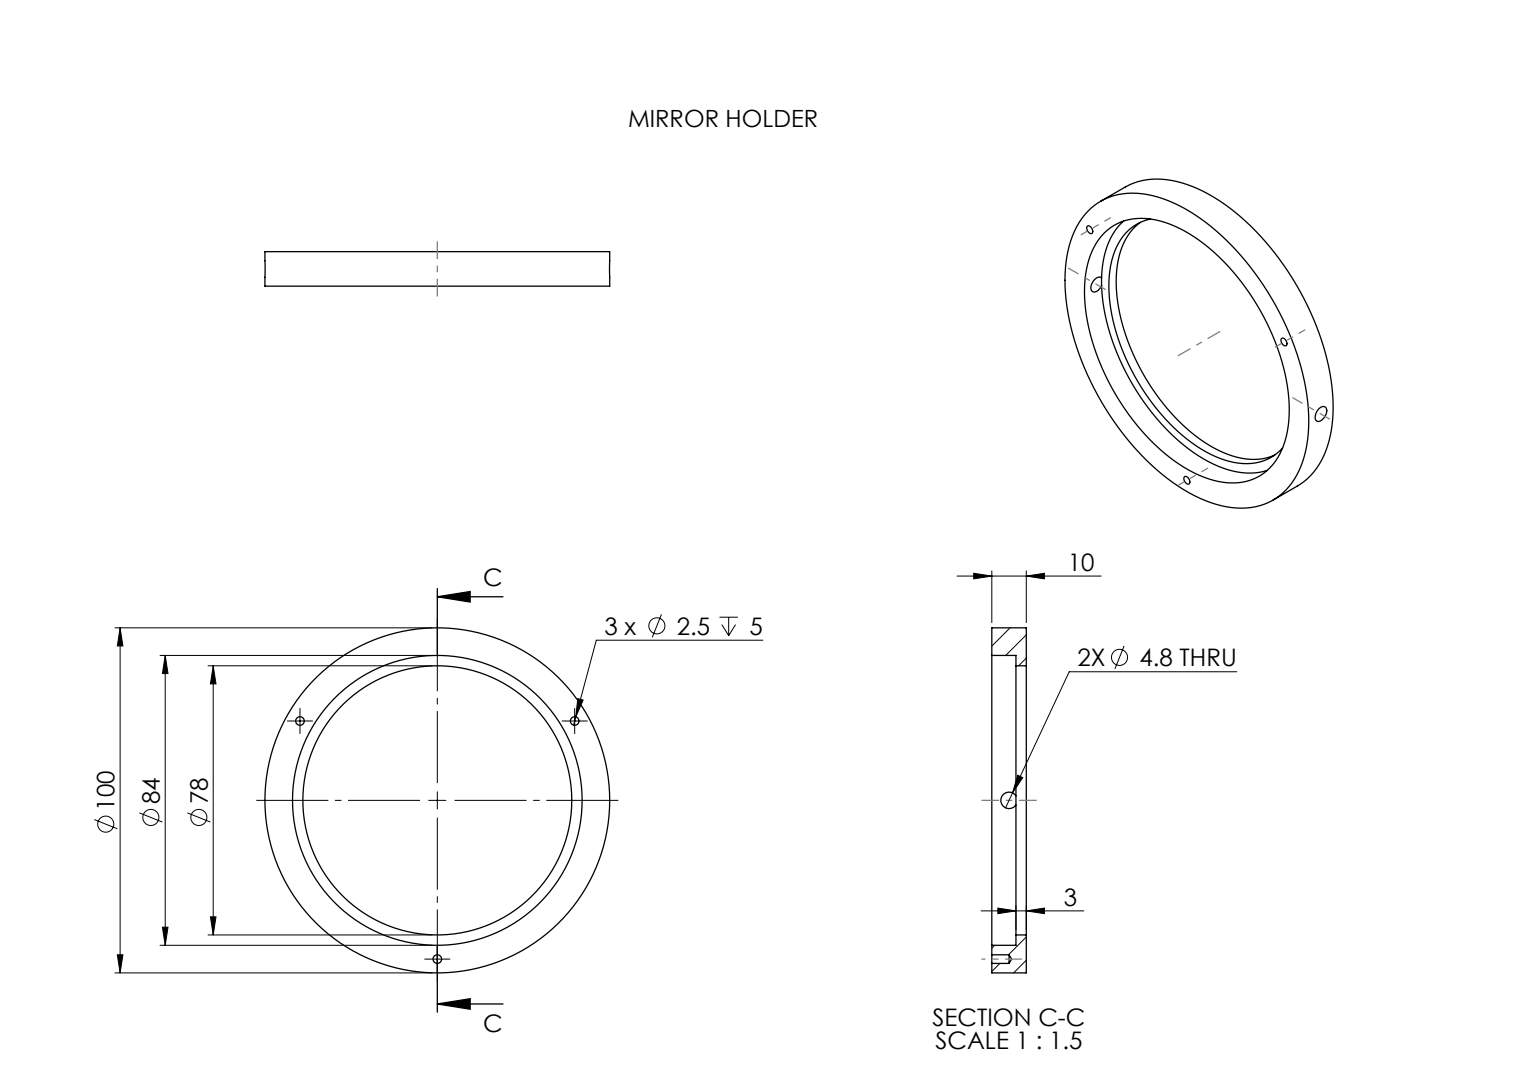
ISO-10303-21;
HEADER;
FILE_DESCRIPTION (('STEP AP214'),
    '1' );
FILE_NAME ('mirror holder.step',
    '2026-10-08T12:12:07',
    ( '' ),
    ( '' ),
    'SwSTEP 2.0',
    'SolidWorks 2026',
    '' );
FILE_SCHEMA (( 'AUTOMOTIVE_DESIGN' ));
ENDSEC;

DATA;
#6=DIRECTION ( 'NONE',  ( -1.000000000000000000, 0.000000000000000000, 0.000000000000000000 ) ) ;
#14=CARTESIAN_POINT ( 'NONE',  ( 49.97494079589864668, 83.41331875350536507, -1.807471472119508205 ) ) ;
#19=CARTESIAN_POINT ( 'NONE',  ( 42.00000000000004263, 84.74554347572708934, -2.399999999999959943 ) ) ;
#22=CYLINDRICAL_SURFACE ( 'NONE', #7576, 2.399999999999985256 ) ;
#23=ORIENTED_EDGE ( 'NONE', *, *, #1900, .T. ) ;
#31=VECTOR ( 'NONE', #6228, 1000.000000000000000 ) ;
#34=FACE_OUTER_BOUND ( 'NONE', #4042, .T. ) ;
#42=ORIENTED_EDGE ( 'NONE', *, *, #1737, .T. ) ;
#44=CARTESIAN_POINT ( 'NONE',  ( -42.00000000000000711, 85.00000000000046896, 2.399999999999971045 ) ) ;
#51=ORIENTED_EDGE ( 'NONE', *, *, #3552, .T. ) ;
#55=CARTESIAN_POINT ( 'NONE',  ( 41.93508307841050708, 82.66544186248239612, -0.5710001583723857133 ) ) ;
#57=ORIENTED_EDGE ( 'NONE', *, *, #5357, .F. ) ;
#58=DIRECTION ( 'NONE',  ( 1.412205397084881070E-17, -2.775557561562891967E-17, -1.000000000000000000 ) ) ;
#59=DIRECTION ( 'NONE',  ( -1.412205397084881070E-17, 2.775557561562891967E-17, 1.000000000000000000 ) ) ;
#71=B_SPLINE_CURVE_WITH_KNOTS ( 'NONE', 3,
 ( #3365, #3998, #818, #3718, #2730, #6286, #158, #589, #14, #5859, #6912, #2467, #2700, #6512, #1264, #1222, #4609, #1172, #6467, #3136, #4426, #5671, #1897, #8185, #2045, #5894, #631, #5007, #778, #5278, #552, #5630 ),
 .UNSPECIFIED., .F., .F.,
 ( 4, 2, 2, 2, 2, 2, 2, 2, 2, 2, 2, 2, 2, 2, 2, 4 ),
 ( 0.000000000000000000, 0.0004690358444888099608, 0.0009380716889776199215, 0.001407107533466429774, 0.001876143377955239843, 0.002345179222444049912, 0.002814215066932859548, 0.003752286755910464074, 0.004221322600399265469, 0.004690358444888067732, 0.005159394289376869995, 0.005628430133865671391, 0.006097465978354474521, 0.006566501822843276784, 0.007035537667332079914, 0.007504573511820881310 ),
 .UNSPECIFIED. ) ;
#72=ORIENTED_EDGE ( 'NONE', *, *, #716, .T. ) ;
#89=CARTESIAN_POINT ( 'NONE',  ( 41.93506701445378582, 87.33484857940398172, -0.5699281247695300312 ) ) ;
#90=DIRECTION ( 'NONE',  ( 0.000000000000000000, 0.000000000000000000, 1.000000000000000000 ) ) ;
#94=( GEOMETRIC_REPRESENTATION_CONTEXT ( 3 ) GLOBAL_UNCERTAINTY_ASSIGNED_CONTEXT ( ( #5253 ) ) GLOBAL_UNIT_ASSIGNED_CONTEXT ( ( #2108, #1487, #1650 ) ) REPRESENTATION_CONTEXT ( 'NONE', 'WORKASPACE' ) );
#108=AXIS2_PLACEMENT_3D ( 'NONE', #7357, #7319, #2957 ) ;
#116=AXIS2_PLACEMENT_3D ( 'NONE', #2904, #405, #2981 ) ;
#126=CARTESIAN_POINT ( 'NONE',  ( 39.00000000000003553, 85.00000000000017053, 2.000000000000043965 ) ) ;
#127=DIRECTION ( 'NONE',  ( -1.000000000000000000, 0.000000000000000000, 2.065146995210483462E-17 ) ) ;
#128=AXIS2_PLACEMENT_3D ( 'NONE', #4289, #6814, #1125 ) ;
#134=ORIENTED_EDGE ( 'NONE', *, *, #338, .F. ) ;
#138=CARTESIAN_POINT ( 'NONE',  ( 41.93122696811919070, 82.59745623955464566, -0.06342023833154092349 ) ) ;
#144=CARTESIAN_POINT ( 'NONE',  ( 5.930697612239895941E-15, 38.99999999999999289, -4.999999999999990230 ) ) ;
#146=CARTESIAN_POINT ( 'NONE',  ( -50.00000000000000711, 85.00000000000009948, -2.399999999999999467 ) ) ;
#150=EDGE_CURVE ( 'NONE', #5220, #7241, #7933, .T. ) ;
#152=CYLINDRICAL_SURFACE ( 'NONE', #1717, 39.00000000000002132 ) ;
#155=CARTESIAN_POINT ( 'NONE',  ( -50.00000000000000711, 85.00000000000009948, 5.000000000000045297 ) ) ;
#158=CARTESIAN_POINT ( 'NONE',  ( 49.98571321592399386, 83.79770962390523437, -2.083050663831888638 ) ) ;
#166=VERTEX_POINT ( 'NONE', #1074 ) ;
#176=DIRECTION ( 'NONE',  ( -1.000000000000000000, 0.000000000000000000, 1.412205397084726379E-17 ) ) ;
#192=ORIENTED_EDGE ( 'NONE', *, *, #1370, .F. ) ;
#201=EDGE_CURVE ( 'NONE', #2355, #5862, #1579, .T. ) ;
#202=DIRECTION ( 'NONE',  ( -1.000000000000000000, 0.000000000000000000, 1.032573497605241731E-17 ) ) ;
#213=STYLED_ITEM ( 'NONE', ( #3872 ), #6686 ) ;
#223=AXIS2_PLACEMENT_3D ( 'NONE', #6794, #1143, #8202 ) ;
#224=CARTESIAN_POINT ( 'NONE',  ( 41.97904239022140160, 83.67335008385828132, 2.000000000000015543 ) ) ;
#231=CIRCLE ( 'NONE', #4093, 50.00000000000002132 ) ;
#242=VECTOR ( 'NONE', #527, 1000.000000000000000 ) ;
#255=DIRECTION ( 'NONE',  ( 1.412205397084881070E-17, -2.775557561562891967E-17, -1.000000000000000000 ) ) ;
#278=DIRECTION ( 'NONE',  ( -1.000000000000000000, 0.000000000000000000, 0.000000000000000000 ) ) ;
#285=DIRECTION ( 'NONE',  ( 1.412205397084881070E-17, -2.775557561562891967E-17, -1.000000000000000000 ) ) ;
#296=FACE_OUTER_BOUND ( 'NONE', #3886, .T. ) ;
#306=CARTESIAN_POINT ( 'NONE',  ( -41.93238906222609330, 87.38229022169096538, 0.3178396967578642762 ) ) ;
#308=CARTESIAN_POINT ( 'NONE',  ( -49.94312129582967685, 82.61555530433810191, -0.3147289805187312162 ) ) ;
#310=FACE_BOUND ( 'NONE', #6643, .T. ) ;
#338=EDGE_CURVE ( 'NONE', #4916, #3085, #3906, .T. ) ;
#358=DIRECTION ( 'NONE',  ( 1.412205397084881070E-17, -2.775557561562891967E-17, -1.000000000000000000 ) ) ;
#363=AXIS2_PLACEMENT_3D ( 'NONE', #6847, #4450, #6938 ) ;
#373=AXIS2_PLACEMENT_3D ( 'NONE', #144, #3901, #4524 ) ;
#376=EDGE_LOOP ( 'NONE', ( #2346, #2970, #7740, #5830, #3828 ) ) ;
#377=AXIS2_PLACEMENT_3D ( 'NONE', #2206, #6560, #5374 ) ;
#392=CARTESIAN_POINT ( 'NONE',  ( -41.94721337724058685, 87.11014508430733372, -1.171319538143981820 ) ) ;
#403=ORIENTED_EDGE ( 'NONE', *, *, #5324, .F. ) ;
#405=DIRECTION ( 'NONE',  ( 1.412205397084881070E-17, -2.775557561562891967E-17, -1.000000000000000000 ) ) ;
#406=CARTESIAN_POINT ( 'NONE',  ( 1.270137496355039850E-14, 85.00000000000011369, 5.000000000000046185 ) ) ;
#411=EDGE_LOOP ( 'NONE', ( #6737, #422 ) ) ;
#419=ADVANCED_FACE ( 'NONE', ( #34 ), #2003, .T. ) ;
#422=ORIENTED_EDGE ( 'NONE', *, *, #7110, .F. ) ;
#423=CARTESIAN_POINT ( 'NONE',  ( 41.98518000931063199, 86.13243788719030647, 2.128825685961691416 ) ) ;
#425=SURFACE_SIDE_STYLE ('',( #7498 ) ) ;
#428=CARTESIAN_POINT ( 'NONE',  ( 50.00000000000002842, 85.15661249647209274, 2.399999999999996803 ) ) ;
#440=ORIENTED_EDGE ( 'NONE', *, *, #4363, .T. ) ;
#467=CARTESIAN_POINT ( 'NONE',  ( -41.93122500247569917, 82.59742185927619573, -0.06338927685520805155 ) ) ;
#468=( LENGTH_UNIT ( ) NAMED_UNIT ( * ) SI_UNIT ( .MILLI., .METRE. ) );
#479=VERTEX_POINT ( 'NONE', #3947 ) ;
#486=CARTESIAN_POINT ( 'NONE',  ( 1.274374112546295138E-14, 85.00000000000017053, 2.000000000000043521 ) ) ;
#493=VERTEX_POINT ( 'NONE', #7205 ) ;
#509=APPLICATION_CONTEXT ( 'automotive_design' ) ;
#513=CARTESIAN_POINT ( 'NONE',  ( -41.96846535023715319, 83.37031242132569275, -1.766478104244469272 ) ) ;
#518=ORIENTED_EDGE ( 'NONE', *, *, #6030, .F. ) ;
#527=DIRECTION ( 'NONE',  ( 1.412205397084881070E-17, -2.775557561562891967E-17, -1.000000000000000000 ) ) ;
#544=EDGE_LOOP ( 'NONE', ( #2163, #4537, #4576, #1786, #8039 ) ) ;
#552=CARTESIAN_POINT ( 'NONE',  ( 50.00000000000001421, 84.84335183244012057, 2.399999999999947509 ) ) ;
#557=CARTESIAN_POINT ( 'NONE',  ( -41.93910753963083948, 82.73888917238660667, -0.8146863085833027096 ) ) ;
#559=AXIS2_PLACEMENT_3D ( 'NONE', #4730, #358, #1076 ) ;
#570=PRODUCT_DEFINITION_FORMATION_WITH_SPECIFIED_SOURCE ( 'ANY', '', #3129, .NOT_KNOWN. ) ;
#578=CARTESIAN_POINT ( 'NONE',  ( 49.94601516505094452, 87.32303837806216507, 0.6228612347032452812 ) ) ;
#589=CARTESIAN_POINT ( 'NONE',  ( 49.97875682971463362, 83.53682071867390846, -1.908850074583744671 ) ) ;
#597=CARTESIAN_POINT ( 'NONE',  ( -41.96116023364841396, 83.19196313526902031, -1.583454828100236522 ) ) ;
#601=DIRECTION ( 'NONE',  ( 1.000000000000000000, 2.775557561562890365E-16, -1.734723475976806478E-17 ) ) ;
#611=B_SPLINE_CURVE_WITH_KNOTS ( 'NONE', 3,
 ( #7772, #6525, #3415, #4045, #1545, #3464 ),
 .UNSPECIFIED., .F., .F.,
 ( 4, 2, 4 ),
 ( 1.267684120349605325E-16, 0.0006999373991970426947, 0.001399874798393958755 ),
 .UNSPECIFIED. ) ;
#617=VECTOR ( 'NONE', #6433, 1000.000000000000114 ) ;
#619=EDGE_LOOP ( 'NONE', ( #2495, #2179, #7102, #6725 ) ) ;
#620=EDGE_CURVE ( 'NONE', #2013, #3227, #3446, .T. ) ;
#626=CARTESIAN_POINT ( 'NONE',  ( -41.98522237648275279, 83.86890273273840535, 2.129714952619055524 ) ) ;
#631=CARTESIAN_POINT ( 'NONE',  ( 49.98889375043669503, 83.93620601285596194, 2.157108981641731038 ) ) ;
#632=AXIS2_PLACEMENT_3D ( 'NONE', #7048, #58, #176 ) ;
#638=CARTESIAN_POINT ( 'NONE',  ( 41.98256188053848348, 83.77272253665795176, -2.078089480949315782 ) ) ;
#654=AXIS2_PLACEMENT_3D ( 'NONE', #1822, #7421, #1144 ) ;
#656=CARTESIAN_POINT ( 'NONE',  ( -50.00000000000000000, 85.31712395750685118, 2.400000000000064748 ) ) ;
#659=CIRCLE ( 'NONE', #7419, 42.00000000000002132 ) ;
#666=CARTESIAN_POINT ( 'NONE',  ( 49.97864901397263537, 86.46689848149799218, -1.906053348878814724 ) ) ;
#667=EDGE_CURVE ( 'NONE', #3060, #2355, #3891, .T. ) ;
#685=CARTESIAN_POINT ( 'NONE',  ( 41.95055335361874427, 82.96164397218471720, 1.273332678597350442 ) ) ;
#686=CARTESIAN_POINT ( 'NONE',  ( 39.00000000000003553, 85.00000000000017053, 5.000000000000047073 ) ) ;
#693=CARTESIAN_POINT ( 'NONE',  ( -49.95346081399732441, 87.15763333356271403, 1.062739361928057402 ) ) ;
#696=CARTESIAN_POINT ( 'NONE',  ( -50.00000000000000711, 85.00000000000009948, 5.000000000000047073 ) ) ;
#703=CARTESIAN_POINT ( 'NONE',  ( -49.97494079589861826, 83.41331875350518033, 1.807471472119332567 ) ) ;
#714=ORIENTED_EDGE ( 'NONE', *, *, #6444, .T. ) ;
#716=EDGE_CURVE ( 'NONE', #4997, #7730, #6980, .T. ) ;
#720=CARTESIAN_POINT ( 'NONE',  ( 41.97904239022140160, 83.67335008385828132, 2.000000000000015543 ) ) ;
#721=CARTESIAN_POINT ( 'NONE',  ( -59.99999999999999289, 85.00000000000045475, -1.387778780781445676E-14 ) ) ;
#732=CARTESIAN_POINT ( 'NONE',  ( 1.274374112546295138E-14, 85.00000000000017053, 2.000000000000043521 ) ) ;
#744=CARTESIAN_POINT ( 'NONE',  ( -42.00000000000000711, 85.00000000000011369, 2.000000000000043077 ) ) ;
#750=CARTESIAN_POINT ( 'NONE',  ( 41.96846535023716029, 86.62968757867487568, -1.766478104244785019 ) ) ;
#766=VECTOR ( 'NONE', #3845, 1000.000000000000000 ) ;
#778=CARTESIAN_POINT ( 'NONE',  ( 49.99635120648666486, 84.37668793019700786, 2.322944911472403451 ) ) ;
#790=CIRCLE ( 'NONE', #7560, 1.249999999999998668 ) ;
#795=AXIS2_PLACEMENT_3D ( 'NONE', #7855, #7230, #6693 ) ;
#798=CARTESIAN_POINT ( 'NONE',  ( 41.99105870351832692, 85.87498856589500917, -2.238438502733319790 ) ) ;
#807=CARTESIAN_POINT ( 'NONE',  ( -49.96357426530714463, 86.91018610273380318, 1.461418215542231058 ) ) ;
#818=CARTESIAN_POINT ( 'NONE',  ( 49.99924596088972351, 84.68545893936931179, -2.384433782424402182 ) ) ;
#820=EDGE_CURVE ( 'NONE', #7254, #5786, #2484, .T. ) ;
#829=ORIENTED_EDGE ( 'NONE', *, *, #2070, .F. ) ;
#842=CYLINDRICAL_SURFACE ( 'NONE', #373, 1.249999999999998446 ) ;
#844=FACE_OUTER_BOUND ( 'NONE', #6718, .T. ) ;
#872=CARTESIAN_POINT ( 'NONE',  ( 39.83716857408421674, 108.0000000000001421, 4.163336342344337027E-14 ) ) ;
#891=AXIS2_PLACEMENT_3D ( 'NONE', #5078, #7003, #1821 ) ;
#910=VERTEX_POINT ( 'NONE', #6172 ) ;
#913=CYLINDRICAL_SURFACE ( 'NONE', #7698, 50.00000000000002132 ) ;
#930=ORIENTED_EDGE ( 'NONE', *, *, #2930, .F. ) ;
#935=CARTESIAN_POINT ( 'NONE',  ( -41.93355926540179723, 87.36154593934628565, -0.4466446237679141396 ) ) ;
#940=LINE ( 'NONE', #5970, #5532 ) ;
#956=CARTESIAN_POINT ( 'NONE',  ( 50.00000000000003553, 85.00000000000012790, 5.000000000000047073 ) ) ;
#958=FACE_OUTER_BOUND ( 'NONE', #3987, .T. ) ;
#977=CARTESIAN_POINT ( 'NONE',  ( -41.95055335361870164, 87.03835602781624914, 1.273332678597377310 ) ) ;
#979=CARTESIAN_POINT ( 'NONE',  ( -49.95347202886236460, 82.84263588727921501, 1.063116165656198264 ) ) ;
#982=CARTESIAN_POINT ( 'NONE',  ( -42.00000000000000711, 85.00000000000011369, -2.399999999999999911 ) ) ;
#993=ORIENTED_EDGE ( 'NONE', *, *, #5499, .F. ) ;
#1001=CIRCLE ( 'NONE', #4066, 1.250000000000001110 ) ;
#1002=B_SPLINE_CURVE_WITH_KNOTS ( 'NONE', 3,
 ( #8152, #3001, #1732, #6920, #3636, #6787, #6161, #1814, #1135, #467, #5548, #4933, #6868, #557, #3677, #1180, #5638, #3772, #597, #513, #1772, #3140, #3052, #8114, #3729, #2433, #2303, #6251 ),
 .UNSPECIFIED., .F., .F.,
 ( 4, 2, 2, 2, 2, 2, 2, 2, 2, 2, 2, 2, 2, 4 ),
 ( 3.925231146709437917E-17, 0.0007633435184944741209, 0.001526687036988908994, 0.001908358796236126051, 0.002290030555483343541, 0.002671702314730560381, 0.003053374073977777655, 0.003435045833224994929, 0.003816717592472212203, 0.004198389351719429910, 0.004580061110966647184, 0.004961732870213864457, 0.005343404629461081731, 0.006106748147955515411 ),
 .UNSPECIFIED. ) ;
#1015=CARTESIAN_POINT ( 'NONE',  ( 41.08716857408421674, 108.0000000000001421, 4.161571085597980959E-14 ) ) ;
#1016=CARTESIAN_POINT ( 'NONE',  ( -41.97904239022133055, 86.32664991614245764, 2.000000000000043521 ) ) ;
#1048=ORIENTED_EDGE ( 'NONE', *, *, #8164, .F. ) ;
#1056=DIRECTION ( 'NONE',  ( 1.412205397084881070E-17, -2.775557561562891967E-17, -1.000000000000000000 ) ) ;
#1065=CARTESIAN_POINT ( 'NONE',  ( -49.98566918070725507, 83.79593159430156390, -2.081985610399898157 ) ) ;
#1070=ADVANCED_FACE ( 'NONE', ( #4597, #7827, #3384, #5307, #2141 ), #6617, .F. ) ;
#1074=CARTESIAN_POINT ( 'NONE',  ( 41.97904239022138029, 86.32664991614251448, 2.000000000000043521 ) ) ;
#1076=DIRECTION ( 'NONE',  ( -1.000000000000000000, 0.000000000000000000, 1.032573497605241731E-17 ) ) ;
#1080=ORIENTED_EDGE ( 'NONE', *, *, #6298, .T. ) ;
#1081=VERTEX_POINT ( 'NONE', #7286 ) ;
#1086=CIRCLE ( 'NONE', #559, 42.00000000000002132 ) ;
#1094=CYLINDRICAL_SURFACE ( 'NONE', #4649, 1.250000000000001110 ) ;
#1098=ADVANCED_FACE ( 'NONE', ( #844 ), #7167, .F. ) ;
#1103=CARTESIAN_POINT ( 'NONE',  ( -42.00000000000001421, 85.25445652427316645, -2.400000000000036326 ) ) ;
#1105=LINE ( 'NONE', #1196, #6872 ) ;
#1113=LINE ( 'NONE', #7561, #7414 ) ;
#1121=ORIENTED_EDGE ( 'NONE', *, *, #3316, .F. ) ;
#1125=DIRECTION ( 'NONE',  ( -1.000000000000000000, 0.000000000000000000, 1.412205397084881070E-17 ) ) ;
#1135=CARTESIAN_POINT ( 'NONE',  ( -41.93161960896017604, 82.60431869815872119, 0.1926422142525844872 ) ) ;
#1143=DIRECTION ( 'NONE',  ( 1.000000000000000000, 1.502586498047605218E-16, -1.412205397084881070E-17 ) ) ;
#1144=DIRECTION ( 'NONE',  ( -1.000000000000000000, 0.000000000000000000, 1.412205397084726379E-17 ) ) ;
#1164=CARTESIAN_POINT ( 'NONE',  ( 1.250000000000003997, 38.99999999999999289, 1.765256746356098409E-17 ) ) ;
#1170=AXIS2_PLACEMENT_3D ( 'NONE', #3288, #7106, #278 ) ;
#1172=CARTESIAN_POINT ( 'NONE',  ( 49.94600989915087297, 82.67684773840547052, 0.6225708050466158827 ) ) ;
#1178=AXIS2_PLACEMENT_3D ( 'NONE', #3683, #6835, #2439 ) ;
#1180=CARTESIAN_POINT ( 'NONE',  ( -41.94739886896328329, 82.89789273483425802, -1.165086683815163449 ) ) ;
#1190=ORIENTED_EDGE ( 'NONE', *, *, #7346, .T. ) ;
#1196=CARTESIAN_POINT ( 'NONE',  ( 42.00000000000003553, 85.00000000000012790, 5.000000000000045297 ) ) ;
#1210=ORIENTED_EDGE ( 'NONE', *, *, #4128, .T. ) ;
#1222=CARTESIAN_POINT ( 'NONE',  ( 49.94236411077207549, 82.59994436935576800, 0.1557065084606094330 ) ) ;
#1223=EDGE_LOOP ( 'NONE', ( #7509, #3451, #6070, #8010 ) ) ;
#1249=( GEOMETRIC_REPRESENTATION_CONTEXT ( 3 ) GLOBAL_UNCERTAINTY_ASSIGNED_CONTEXT ( ( #6118 ) ) GLOBAL_UNIT_ASSIGNED_CONTEXT ( ( #1271, #6870, #1733 ) ) REPRESENTATION_CONTEXT ( 'NONE', 'WORKASPACE' ) );
#1251=CARTESIAN_POINT ( 'NONE',  ( 49.96366046868875088, 86.90794461356699685, 1.464368789227024736 ) ) ;
#1256=PRODUCT_DEFINITION_CONTEXT ( 'detailed design', #509, 'design' ) ;
#1259=CARTESIAN_POINT ( 'NONE',  ( -41.99795150464620974, 84.52878598459807336, 2.364843771231078584 ) ) ;
#1264=CARTESIAN_POINT ( 'NONE',  ( 49.94237215279112263, 82.60011171831010302, -0.3139783802612605146 ) ) ;
#1265=ORIENTED_EDGE ( 'NONE', *, *, #1900, .F. ) ;
#1267=LINE ( 'NONE', #7624, #4912 ) ;
#1268=CARTESIAN_POINT ( 'NONE',  ( 41.97224931050730845, 83.45839738397258145, 1.857416509361046630 ) ) ;
#1270=ADVANCED_FACE ( 'NONE', ( #1773 ), #1094, .F. ) ;
#1271=( LENGTH_UNIT ( ) NAMED_UNIT ( * ) SI_UNIT ( .MILLI., .METRE. ) );
#1284=CARTESIAN_POINT ( 'NONE',  ( -49.99683717277851258, 85.63216245974585661, 2.336254100262071809 ) ) ;
#1296=CARTESIAN_POINT ( 'NONE',  ( 41.99057456900149532, 84.08235334355106261, 2.230005891995792133 ) ) ;
#1310=CARTESIAN_POINT ( 'NONE',  ( 41.93910753963084659, 87.26111082761428861, -0.8146863085835460705 ) ) ;
#1329=CARTESIAN_POINT ( 'NONE',  ( -39.00000000000000711, 85.00000000000017053, 5.000000000000045297 ) ) ;
#1333=DIRECTION ( 'NONE',  ( -1.000000000000000000, 0.000000000000000000, 2.065146995210483462E-17 ) ) ;
#1340=ADVANCED_FACE ( 'NONE', ( #7539 ), #22, .F. ) ;
#1350=EDGE_CURVE ( 'NONE', #4097, #5106, #4928, .T. ) ;
#1358=CARTESIAN_POINT ( 'NONE',  ( 41.93162413031729585, 82.60433940584233881, -0.1928755069450422688 ) ) ;
#1359=CYLINDRICAL_SURFACE ( 'NONE', #7664, 2.399999999999985256 ) ;
#1370=EDGE_CURVE ( 'NONE', #5556, #3085, #2015, .T. ) ;
#1371=CARTESIAN_POINT ( 'NONE',  ( -49.98886144361672734, 86.06516230458035466, 2.156352803700620768 ) ) ;
#1376=DIRECTION ( 'NONE',  ( 1.000000000000000000, 0.000000000000000000, -1.112002228190260397E-17 ) ) ;
#1398=LINE ( 'NONE', #7743, #5160 ) ;
#1406=CARTESIAN_POINT ( 'NONE',  ( -49.94817596271295201, 87.27669880683387760, -0.7754554817172341075 ) ) ;
#1416=ADVANCED_FACE ( 'NONE', ( #7818 ), #7120, .F. ) ;
#1427=PRODUCT_DEFINITION ( 'UNKNOWN', '', #570, #1256 ) ;
#1429=VERTEX_POINT ( 'NONE', #4670 ) ;
#1432=CARTESIAN_POINT ( 'NONE',  ( 41.94112359463814954, 82.77568671679536294, -0.9366119428080386111 ) ) ;
#1444=CIRCLE ( 'NONE', #5554, 1.249999999999998668 ) ;
#1447=EDGE_LOOP ( 'NONE', ( #6676, #192 ) ) ;
#1464=DIRECTION ( 'NONE',  ( -0.8571673007021118895, -1.430919794933844670E-16, -0.5150380749100549327 ) ) ;
#1466=EDGE_CURVE ( 'NONE', #7254, #493, #7769, .T. ) ;
#1481=DIRECTION ( 'NONE',  ( 1.412205397084881070E-17, -2.775557561562891967E-17, -1.000000000000000000 ) ) ;
#1483=DIRECTION ( 'NONE',  ( -1.000000000000000000, -1.502586498047605218E-16, 1.238733049487200360E-17 ) ) ;
#1487=( NAMED_UNIT ( * ) PLANE_ANGLE_UNIT ( ) SI_UNIT ( $, .RADIAN. ) );
#1497=ORIENTED_EDGE ( 'NONE', *, *, #7301, .T. ) ;
#1502=FACE_OUTER_BOUND ( 'NONE', #6197, .T. ) ;
#1512=DIRECTION ( 'NONE',  ( 1.412205397084881070E-17, -2.775557561562891967E-17, -1.000000000000000000 ) ) ;
#1515=DIRECTION ( 'NONE',  ( -1.000000000000000000, 0.000000000000000000, 0.000000000000000000 ) ) ;
#1517=CARTESIAN_POINT ( 'NONE',  ( -59.99999999999999289, 85.00000000000045475, -1.387778780781445676E-14 ) ) ;
#1536=LINE ( 'NONE', #6474, #4626 ) ;
#1545=CARTESIAN_POINT ( 'NONE',  ( -41.98520465537847457, 86.13165801428257851, 2.129342995125455662 ) ) ;
#1553=ADVANCED_FACE ( 'NONE', ( #5418 ), #7935, .T. ) ;
#1559=ORIENTED_EDGE ( 'NONE', *, *, #7278, .F. ) ;
#1561=CONICAL_SURFACE ( 'NONE', #3019, 1.249999999999998002, 1.029744258676653645 ) ;
#1566=ADVANCED_FACE ( 'NONE', ( #1641 ), #6697, .F. ) ;
#1569=CIRCLE ( 'NONE', #363, 50.00000000000002132 ) ;
#1579=CIRCLE ( 'NONE', #5829, 42.00000000000002132 ) ;
#1587=AXIS2_PLACEMENT_3D ( 'NONE', #3942, #5152, #6454 ) ;
#1598=EDGE_CURVE ( 'NONE', #5786, #1081, #7237, .T. ) ;
#1600=DIRECTION ( 'NONE',  ( -1.000000000000000000, 0.000000000000000000, 0.000000000000000000 ) ) ;
#1601=CIRCLE ( 'NONE', #795, 39.00000000000002132 ) ;
#1622=DIRECTION ( 'NONE',  ( 1.000000000000000000, 1.502586498047605218E-16, -1.412205397084881070E-17 ) ) ;
#1630=EDGE_CURVE ( 'NONE', #7075, #7290, #71, .T. ) ;
#1641=FACE_OUTER_BOUND ( 'NONE', #2635, .T. ) ;
#1647=EDGE_CURVE ( 'NONE', #7219, #5129, #1001, .T. ) ;
#1650=( NAMED_UNIT ( * ) SI_UNIT ( $, .STERADIAN. ) SOLID_ANGLE_UNIT ( ) );
#1654=CARTESIAN_POINT ( 'NONE',  ( -49.99423685432763875, 84.22705925652886094, -2.277573141052998462 ) ) ;
#1671=DIRECTION ( 'NONE',  ( 1.000000000000000000, 1.502586498047605218E-16, -1.412205397084881070E-17 ) ) ;
#1672=CARTESIAN_POINT ( 'NONE',  ( -41.08716857408418122, 108.0000000000001990, -4.999999999999976907 ) ) ;
#1687=ORIENTED_EDGE ( 'NONE', *, *, #7096, .T. ) ;
#1692=CARTESIAN_POINT ( 'NONE',  ( -41.97904239022133055, 86.32664991614245764, 2.000000000000043521 ) ) ;
#1711=EDGE_LOOP ( 'NONE', ( #4384, #23, #2821 ) ) ;
#1717=AXIS2_PLACEMENT_3D ( 'NONE', #732, #5741, #1376 ) ;
#1726=AXIS2_PLACEMENT_3D ( 'NONE', #5818, #5131, #6438 ) ;
#1732=CARTESIAN_POINT ( 'NONE',  ( -41.96471864142489494, 83.27150586048362868, 1.684781847096441298 ) ) ;
#1733=( NAMED_UNIT ( * ) SI_UNIT ( $, .STERADIAN. ) SOLID_ANGLE_UNIT ( ) );
#1737=EDGE_CURVE ( 'NONE', #1769, #4916, #940, .T. ) ;
#1742=CYLINDRICAL_SURFACE ( 'NONE', #223, 2.399999999999985256 ) ;
#1744=DIRECTION ( 'NONE',  ( 1.412205397084881070E-17, -2.775557561562891967E-17, -1.000000000000000000 ) ) ;
#1756=CARTESIAN_POINT ( 'NONE',  ( 49.94311118432961649, 87.38465289139496406, -0.3128412141714160266 ) ) ;
#1762=DIRECTION ( 'NONE',  ( 1.412205397084881070E-17, -2.775557561562891967E-17, -1.000000000000000000 ) ) ;
#1764=FACE_OUTER_BOUND ( 'NONE', #2988, .T. ) ;
#1767=DIRECTION ( 'NONE',  ( -1.000000000000000000, 0.000000000000000000, 2.065146995210483462E-17 ) ) ;
#1769=VERTEX_POINT ( 'NONE', #982 ) ;
#1772=CARTESIAN_POINT ( 'NONE',  ( -41.97210380486418302, 83.46605959390291218, -1.850206309317909303 ) ) ;
#1773=FACE_OUTER_BOUND ( 'NONE', #6146, .T. ) ;
#1786=ORIENTED_EDGE ( 'NONE', *, *, #4520, .T. ) ;
#1792=CARTESIAN_POINT ( 'NONE',  ( -39.00000000000000711, 85.00000000000017053, 2.000000000000043965 ) ) ;
#1793=DIRECTION ( 'NONE',  ( -1.412205397084881070E-17, 2.775557561562891967E-17, 1.000000000000000000 ) ) ;
#1800=EDGE_LOOP ( 'NONE', ( #1919, #2477, #6514, #4664 ) ) ;
#1801=ORIENTED_EDGE ( 'NONE', *, *, #3973, .T. ) ;
#1814=CARTESIAN_POINT ( 'NONE',  ( -41.93240078214817856, 82.61791640338877585, 0.3192077737422600037 ) ) ;
#1818=ORIENTED_EDGE ( 'NONE', *, *, #6302, .F. ) ;
#1821=DIRECTION ( 'NONE',  ( -1.000000000000000000, 0.000000000000000000, 1.032573497605241731E-17 ) ) ;
#1822=CARTESIAN_POINT ( 'NONE',  ( -39.83716857408418122, 108.0000000000001421, 4.163336342344337027E-14 ) ) ;
#1834=CARTESIAN_POINT ( 'NONE',  ( 49.99422766321050204, 85.77334557296516948, 2.277359159638543851 ) ) ;
#1861=CARTESIAN_POINT ( 'NONE',  ( -42.00000000000000711, 85.00000000000046896, 2.399999999999971045 ) ) ;
#1864=DIRECTION ( 'NONE',  ( 1.000000000000000000, 2.775557561562890365E-16, -1.734723475976806478E-17 ) ) ;
#1870=CYLINDRICAL_SURFACE ( 'NONE', #5302, 39.00000000000002132 ) ;
#1873=VECTOR ( 'NONE', #1744, 1000.000000000000000 ) ;
#1877=AXIS2_PLACEMENT_3D ( 'NONE', #6386, #5148, #601 ) ;
#1888=CARTESIAN_POINT ( 'NONE',  ( 41.97904239022140160, 83.67335008385828132, 2.000000000000015543 ) ) ;
#1892=FACE_OUTER_BOUND ( 'NONE', #1223, .T. ) ;
#1897=CARTESIAN_POINT ( 'NONE',  ( 49.96737414687255097, 83.19055800108181131, 1.584620125915989775 ) ) ;
#1900=EDGE_CURVE ( 'NONE', #7604, #5220, #7469, .T. ) ;
#1904=CARTESIAN_POINT ( 'NONE',  ( 41.96864087686234512, 83.36448938425077415, -1.774759388939936899 ) ) ;
#1911=ORIENTED_EDGE ( 'NONE', *, *, #6672, .F. ) ;
#1919=ORIENTED_EDGE ( 'NONE', *, *, #1466, .F. ) ;
#1926=CARTESIAN_POINT ( 'NONE',  ( 50.00000000000004974, 85.31712395750716382, -2.400000000000014566 ) ) ;
#1944=CARTESIAN_POINT ( 'NONE',  ( 42.00000000000003553, 85.00000000000012790, -2.399999999999999023 ) ) ;
#1950=DIRECTION ( 'NONE',  ( 1.412205397084881070E-17, -2.775557561562891967E-17, -1.000000000000000000 ) ) ;
#1963=CARTESIAN_POINT ( 'NONE',  ( -49.99924596088969508, 84.68545893936895652, 2.384433782424337789 ) ) ;
#1968=ORIENTED_EDGE ( 'NONE', *, *, #7077, .F. ) ;
#1981=CARTESIAN_POINT ( 'NONE',  ( 41.93161561614421373, 82.60424888756949713, 0.1913511295313893579 ) ) ;
#1997=CARTESIAN_POINT ( 'NONE',  ( -49.94313152867111683, 87.38422970439138737, -0.3160888171752656572 ) ) ;
#2001=ORIENTED_EDGE ( 'NONE', *, *, #7821, .F. ) ;
#2002=AXIS2_PLACEMENT_3D ( 'NONE', #4200, #1762, #6191 ) ;
#2003=CYLINDRICAL_SURFACE ( 'NONE', #6823, 42.00000000000002132 ) ;
#2013=VERTEX_POINT ( 'NONE', #1329 ) ;
#2015=CIRCLE ( 'NONE', #1877, 50.00000000000002132 ) ;
#2017=CARTESIAN_POINT ( 'NONE',  ( -38.58716857408418122, 108.0000000000001990, -4.999999999999976907 ) ) ;
#2025=DIRECTION ( 'NONE',  ( 1.412205397084881070E-17, -2.775557561562891967E-17, -1.000000000000000000 ) ) ;
#2026=CARTESIAN_POINT ( 'NONE',  ( 42.00000000000003553, 85.00000000000012790, -2.399999999999999023 ) ) ;
#2039=DIRECTION ( 'NONE',  ( 1.412205397084881070E-17, -2.775557561562891967E-17, -1.000000000000000000 ) ) ;
#2045=CARTESIAN_POINT ( 'NONE',  ( 49.97873132679187336, 83.53599209938494141, 1.908173386893731616 ) ) ;
#2059=CARTESIAN_POINT ( 'NONE',  ( 41.93240078214817146, 87.38208359661221891, 0.3192077737421512018 ) ) ;
#2064=DIRECTION ( 'NONE',  ( 1.412205397084881070E-17, -2.775557561562891967E-17, -1.000000000000000000 ) ) ;
#2070=EDGE_CURVE ( 'NONE', #4916, #1429, #3080, .T. ) ;
#2079=AXIS2_PLACEMENT_3D ( 'NONE', #6156, #3544, #6821 ) ;
#2102=CIRCLE ( 'NONE', #891, 42.00000000000002132 ) ;
#2104=CIRCLE ( 'NONE', #6349, 42.00000000000002132 ) ;
#2108=( LENGTH_UNIT ( ) NAMED_UNIT ( * ) SI_UNIT ( .MILLI., .METRE. ) );
#2126=VECTOR ( 'NONE', #5355, 1000.000000000000000 ) ;
#2141=FACE_BOUND ( 'NONE', #3104, .T. ) ;
#2149=CARTESIAN_POINT ( 'NONE',  ( -49.95667649488481032, 82.91716997302802383, 1.202799388691194959 ) ) ;
#2163=ORIENTED_EDGE ( 'NONE', *, *, #6444, .F. ) ;
#2173=LINE ( 'NONE', #4130, #7287 ) ;
#2179=ORIENTED_EDGE ( 'NONE', *, *, #2648, .T. ) ;
#2188=CARTESIAN_POINT ( 'NONE',  ( 1.274374112546295138E-14, 85.00000000000017053, 2.000000000000043521 ) ) ;
#2206=CARTESIAN_POINT ( 'NONE',  ( -39.83716857408418122, 108.0000000000001990, -4.999999999999976907 ) ) ;
#2226=CARTESIAN_POINT ( 'NONE',  ( -49.97498335796541369, 83.41456698278581428, -1.808729786019619423 ) ) ;
#2231=ORIENTED_EDGE ( 'NONE', *, *, #5399, .T. ) ;
#2236=AXIS2_PLACEMENT_3D ( 'NONE', #3540, #4202, #6778 ) ;
#2242=CARTESIAN_POINT ( 'NONE',  ( -41.08716857408418122, 108.0000000000001990, -4.999999999999976907 ) ) ;
#2246=PRODUCT_CONTEXT ( 'NONE', #7736, 'mechanical' ) ;
#2255=AXIS2_PLACEMENT_3D ( 'NONE', #4020, #255, #6032 ) ;
#2267=ORIENTED_EDGE ( 'NONE', *, *, #2993, .T. ) ;
#2273=LINE ( 'NONE', #6711, #6943 ) ;
#2302=CARTESIAN_POINT ( 'NONE',  ( 41.97904239022138029, 86.32664991614251448, 2.000000000000043521 ) ) ;
#2303=CARTESIAN_POINT ( 'NONE',  ( -42.00000000000001421, 84.74546678807557498, -2.399999999999965272 ) ) ;
#2308=EDGE_LOOP ( 'NONE', ( #1818, #5430, #1801, #6222, #3675, #134, #6812, #7886 ) ) ;
#2311=CARTESIAN_POINT ( 'NONE',  ( -42.00000000000000711, 85.00000000000011369, -2.399999999999999911 ) ) ;
#2334=DIRECTION ( 'NONE',  ( 1.412205397084881070E-17, -2.775557561562891967E-17, -1.000000000000000000 ) ) ;
#2346=ORIENTED_EDGE ( 'NONE', *, *, #2525, .T. ) ;
#2348=CARTESIAN_POINT ( 'NONE',  ( -41.95400501379501890, 86.96664633062719929, 1.381527937806870998 ) ) ;
#2349=DIRECTION ( 'NONE',  ( -1.000000000000000000, -1.502586498047605218E-16, 1.238733049487200360E-17 ) ) ;
#2350=DIRECTION ( 'NONE',  ( 1.412205397084881070E-17, -2.775557561562891967E-17, -1.000000000000000000 ) ) ;
#2355=VERTEX_POINT ( 'NONE', #224 ) ;
#2363=CARTESIAN_POINT ( 'NONE',  ( -42.00000000000000711, 85.00000000000011369, -5.000000000000005329 ) ) ;
#2373=ORIENTED_EDGE ( 'NONE', *, *, #5785, .T. ) ;
#2386=CIRCLE ( 'NONE', #377, 1.250000000000001110 ) ;
#2389=ADVANCED_FACE ( 'NONE', ( #3444 ), #7320, .F. ) ;
#2396=AXIS2_PLACEMENT_3D ( 'NONE', #2569, #5111, #1864 ) ;
#2433=CARTESIAN_POINT ( 'NONE',  ( -41.99757081983619145, 84.48764332354225814, -2.358461006662856185 ) ) ;
#2439=DIRECTION ( 'NONE',  ( -1.000000000000000000, 0.000000000000000000, 1.412205397084726379E-17 ) ) ;
#2452=DIRECTION ( 'NONE',  ( 1.412205397084881070E-17, -2.775557561562891967E-17, -1.000000000000000000 ) ) ;
#2457=ADVANCED_FACE ( 'NONE', ( #7872, #310 ), #7837, .T. ) ;
#2467=CARTESIAN_POINT ( 'NONE',  ( 49.95667649488486717, 82.91716997302819436, -1.202799388691395910 ) ) ;
#2477=ORIENTED_EDGE ( 'NONE', *, *, #820, .T. ) ;
#2484=LINE ( 'NONE', #6218, #242 ) ;
#2493=CARTESIAN_POINT ( 'NONE',  ( 49.97874610126637407, 86.47445480916304916, 1.919346332466817406 ) ) ;
#2495=ORIENTED_EDGE ( 'NONE', *, *, #7453, .T. ) ;
#2498=ORIENTED_EDGE ( 'NONE', *, *, #7821, .T. ) ;
#2517=CARTESIAN_POINT ( 'NONE',  ( 41.96116023364841396, 86.80803686473167602, -1.583454828100570255 ) ) ;
#2519=PRESENTATION_STYLE_ASSIGNMENT (( #6295 ) ) ;
#2525=EDGE_CURVE ( 'NONE', #166, #2355, #1086, .T. ) ;
#2527=ORIENTED_EDGE ( 'NONE', *, *, #667, .T. ) ;
#2548=CARTESIAN_POINT ( 'NONE',  ( 49.96738998307159818, 86.80892218194638588, -1.585032901986132226 ) ) ;
#2552=CARTESIAN_POINT ( 'NONE',  ( 41.99758845363990645, 84.53527270025752216, 2.357482664457419830 ) ) ;
#2567=AXIS2_PLACEMENT_3D ( 'NONE', #4143, #5319, #4687 ) ;
#2569=CARTESIAN_POINT ( 'NONE',  ( 1.270137496355039850E-14, 85.00000000000011369, 5.000000000000046185 ) ) ;
#2578=CARTESIAN_POINT ( 'NONE',  ( -49.94236053903777162, 87.40012995604533330, 0.1563225272305456826 ) ) ;
#2583=( GEOMETRIC_REPRESENTATION_CONTEXT ( 3 ) GLOBAL_UNCERTAINTY_ASSIGNED_CONTEXT ( ( #8018 ) ) GLOBAL_UNIT_ASSIGNED_CONTEXT ( ( #468, #3002, #5014 ) ) REPRESENTATION_CONTEXT ( 'NONE', 'WORKASPACE' ) );
#2610=CARTESIAN_POINT ( 'NONE',  ( 50.00000000000003553, 85.00000000000012790, 5.000000000000045297 ) ) ;
#2618=LINE ( 'NONE', #7642, #617 ) ;
#2635=EDGE_LOOP ( 'NONE', ( #5794, #6445, #51, #3105 ) ) ;
#2637=CARTESIAN_POINT ( 'NONE',  ( 41.96471864142488073, 86.72849413951723818, 1.684781847096518792 ) ) ;
#2640=VECTOR ( 'NONE', #3843, 1000.000000000000114 ) ;
#2648=EDGE_CURVE ( 'NONE', #4584, #2013, #3077, .T. ) ;
#2654=CARTESIAN_POINT ( 'NONE',  ( -49.97864901397259985, 86.46689848149772217, 1.906053348878929077 ) ) ;
#2661=FACE_OUTER_BOUND ( 'NONE', #8158, .T. ) ;
#2670=ORIENTED_EDGE ( 'NONE', *, *, #2525, .F. ) ;
#2678=CARTESIAN_POINT ( 'NONE',  ( 41.93504501510003735, 82.66492853475577363, 0.5690079308735644936 ) ) ;
#2679=CARTESIAN_POINT ( 'NONE',  ( -39.83716857408418122, 108.0000000000001421, 4.163336342344337027E-14 ) ) ;
#2683=EDGE_CURVE ( 'NONE', #5862, #7730, #6790, .T. ) ;
#2700=CARTESIAN_POINT ( 'NONE',  ( 49.95347202886240012, 82.84263588727935712, -1.063116165656391221 ) ) ;
#2703=MECHANICAL_DESIGN_GEOMETRIC_PRESENTATION_REPRESENTATION('',(#6950),#2583);
#2725=CYLINDRICAL_SURFACE ( 'NONE', #6206, 42.00000000000002132 ) ;
#2730=CARTESIAN_POINT ( 'NONE',  ( 49.99422363137632885, 84.22622254513471773, -2.277283319317807031 ) ) ;
#2746=ORIENTED_EDGE ( 'NONE', *, *, #7323, .F. ) ;
#2753=CARTESIAN_POINT ( 'NONE',  ( 39.83716857408421674, 108.0000000000001990, -4.999999999999976907 ) ) ;
#2758=CYLINDRICAL_SURFACE ( 'NONE', #2255, 1.249999999999998446 ) ;
#2791=ORIENTED_EDGE ( 'NONE', *, *, #5357, .T. ) ;
#2795=DIRECTION ( 'NONE',  ( 1.412205397084881070E-17, -2.775557561562891967E-17, -1.000000000000000000 ) ) ;
#2798=DIRECTION ( 'NONE',  ( 1.412205397084881070E-17, -2.775557561562891967E-17, -1.000000000000000000 ) ) ;
#2813=CARTESIAN_POINT ( 'NONE',  ( -41.94160807294379367, 87.21436019787591931, 0.9342823132686582932 ) ) ;
#2821=ORIENTED_EDGE ( 'NONE', *, *, #150, .T. ) ;
#2841=DIRECTION ( 'NONE',  ( -1.000000000000000000, 0.000000000000000000, 1.412205397084726379E-17 ) ) ;
#2851=DIRECTION ( 'NONE',  ( -1.000000000000000000, 0.000000000000000000, 0.000000000000000000 ) ) ;
#2853=CARTESIAN_POINT ( 'NONE',  ( -49.95669240716469517, 82.91758674606776935, -1.203334160065746339 ) ) ;
#2854=DIRECTION ( 'NONE',  ( -1.000000000000000000, -1.502586498047605218E-16, 1.412205397084881070E-17 ) ) ;
#2868=AXIS2_PLACEMENT_3D ( 'NONE', #3767, #5717, #3332 ) ;
#2874=ORIENTED_EDGE ( 'NONE', *, *, #2683, .F. ) ;
#2891=LINE ( 'NONE', #1015, #4865 ) ;
#2894=CARTESIAN_POINT ( 'NONE',  ( -49.94600989915083744, 82.67684773840545631, -0.6225708050467673171 ) ) ;
#2904=CARTESIAN_POINT ( 'NONE',  ( 5.860087342385653250E-15, 38.99999999999999289, 0.000000000000000000 ) ) ;
#2905=CIRCLE ( 'NONE', #5045, 42.00000000000002132 ) ;
#2918=VECTOR ( 'NONE', #4201, 1000.000000000000000 ) ;
#2920=ORIENTED_EDGE ( 'NONE', *, *, #6168, .F. ) ;
#2925=AXIS2_PLACEMENT_3D ( 'NONE', #1517, #1483, #5345 ) ;
#2930=EDGE_CURVE ( 'NONE', #479, #5129, #2618, .T. ) ;
#2937=CARTESIAN_POINT ( 'NONE',  ( -41.93161561614412847, 87.39575111243146921, 0.1913511295312773086 ) ) ;
#2941=ORIENTED_EDGE ( 'NONE', *, *, #4363, .F. ) ;
#2946=DIRECTION ( 'NONE',  ( 1.000000000000000000, 2.775557561562890365E-16, -1.734723475976806478E-17 ) ) ;
#2957=DIRECTION ( 'NONE',  ( -1.000000000000000000, 0.000000000000000000, 2.065146995210483462E-17 ) ) ;
#2964=CARTESIAN_POINT ( 'NONE',  ( 42.00000000000003553, 85.00000000000049738, 2.399999999999971934 ) ) ;
#2970=ORIENTED_EDGE ( 'NONE', *, *, #201, .T. ) ;
#2973=CARTESIAN_POINT ( 'NONE',  ( -41.93508307841045024, 87.33455813751852759, -0.5710001583726183050 ) ) ;
#2975=LINE ( 'NONE', #5519, #1873 ) ;
#2981=DIRECTION ( 'NONE',  ( -1.000000000000000000, 0.000000000000000000, 1.412205397084881070E-17 ) ) ;
#2988=EDGE_LOOP ( 'NONE', ( #7756, #8019, #6112, #1210, #7036, #7651, #1121, #3848 ) ) ;
#2993=EDGE_CURVE ( 'NONE', #4127, #7254, #2891, .T. ) ;
#3001=CARTESIAN_POINT ( 'NONE',  ( -41.97224725382100274, 83.45833230446734774, 1.857373340501012660 ) ) ;
#3002=( NAMED_UNIT ( * ) PLANE_ANGLE_UNIT ( ) SI_UNIT ( $, .RADIAN. ) );
#3019=AXIS2_PLACEMENT_3D ( 'NONE', #7184, #5174, #7070 ) ;
#3020=ORIENTED_EDGE ( 'NONE', *, *, #4793, .T. ) ;
#3024=DIRECTION ( 'NONE',  ( -1.000000000000000000, 0.000000000000000000, 1.032573497605241731E-17 ) ) ;
#3036=ORIENTED_EDGE ( 'NONE', *, *, #2993, .F. ) ;
#3050=CIRCLE ( 'NONE', #7569, 1.250000000000001110 ) ;
#3052=CARTESIAN_POINT ( 'NONE',  ( -41.98244464128907794, 83.78046611586739800, -2.071021427375471902 ) ) ;
#3060=VERTEX_POINT ( 'NONE', #6577 ) ;
#3073=EDGE_LOOP ( 'NONE', ( #4827, #714, #6402, #6165, #1497 ) ) ;
#3077=LINE ( 'NONE', #1792, #31 ) ;
#3079=CARTESIAN_POINT ( 'NONE',  ( 49.97491191256678178, 86.58758952878010007, -1.806678789609242664 ) ) ;
#3080=B_SPLINE_CURVE_WITH_KNOTS ( 'NONE', 3,
 ( #146, #3869, #5234, #5120, #7089, #6395, #3904, #4598, #6428, #3986, #5082, #1406, #3240, #1997, #4483, #2578, #4528, #6503, #7602, #693, #7052, #807, #6350, #3944, #2654, #6968, #1371, #1284, #656, #3205 ),
 .UNSPECIFIED., .F., .F.,
 ( 4, 2, 2, 2, 2, 2, 2, 2, 2, 2, 2, 2, 2, 2, 4 ),
 ( 0.007504573511820675745, 0.007973502549960232236, 0.008442431588099789594, 0.009380289664378940739, 0.009849218702518501567, 0.01031814774065806413, 0.01078707677879762669, 0.01125600581693718752, 0.01172493485507674835, 0.01219386389321631091, 0.01266279293135587347, 0.01313172196949543430, 0.01360065100763499513, 0.01406958004577455595, 0.01500743812205367934 ),
 .UNSPECIFIED. ) ;
#3085=VERTEX_POINT ( 'NONE', #7867 ) ;
#3086=DIRECTION ( 'NONE',  ( 1.412205397084881070E-17, -2.775557561562891967E-17, -1.000000000000000000 ) ) ;
#3096=CARTESIAN_POINT ( 'NONE',  ( 50.00000000000003553, 85.00000000000012790, 2.399999999999971489 ) ) ;
#3098=FILL_AREA_STYLE_COLOUR ( '', #5883 ) ;
#3104=EDGE_LOOP ( 'NONE', ( #2373, #4277 ) ) ;
#3105=ORIENTED_EDGE ( 'NONE', *, *, #5324, .T. ) ;
#3121=CARTESIAN_POINT ( 'NONE',  ( 49.99637443241782364, 85.62167278847336149, 2.323444847100735178 ) ) ;
#3129=PRODUCT ( 'mirror holder', 'mirror holder', '', ( #2246 ) ) ;
#3136=CARTESIAN_POINT ( 'NONE',  ( 49.95346277782375921, 82.84241399044236687, 1.062802698623439568 ) ) ;
#3140=CARTESIAN_POINT ( 'NONE',  ( -41.97907998747121638, 83.67059623091998333, -2.002229301367134617 ) ) ;
#3162=CARTESIAN_POINT ( 'NONE',  ( 41.08716857408421674, 108.0000000000001990, -4.999999999999976907 ) ) ;
#3164=CARTESIAN_POINT ( 'NONE',  ( 49.94237310791758944, 87.39986840612067454, 0.1602877778558433053 ) ) ;
#3167=AXIS2_PLACEMENT_3D ( 'NONE', #2679, #2798, #3302 ) ;
#3171=CIRCLE ( 'NONE', #632, 1.250000000000001110 ) ;
#3189=CARTESIAN_POINT ( 'NONE',  ( 41.94160807294385762, 82.78563980212508966, 0.9342823132686682852 ) ) ;
#3194=CIRCLE ( 'NONE', #5191, 39.00000000000002132 ) ;
#3196=ORIENTED_EDGE ( 'NONE', *, *, #4960, .T. ) ;
#3205=CARTESIAN_POINT ( 'NONE',  ( -49.99999999999999289, 85.00000000000005684, 2.400000000000013234 ) ) ;
#3213=CARTESIAN_POINT ( 'NONE',  ( 49.94597403161979798, 87.32391958025814915, -0.6195456578939724235 ) ) ;
#3216=DIRECTION ( 'NONE',  ( 1.412205397084881070E-17, -2.775557561562891967E-17, -1.000000000000000000 ) ) ;
#3227=VERTEX_POINT ( 'NONE', #686 ) ;
#3231=CARTESIAN_POINT ( 'NONE',  ( 41.95042219981620235, 87.04630884801559887, 1.280157006458500613 ) ) ;
#3233=AXIS2_PLACEMENT_3D ( 'NONE', #486, #2452, #3024 ) ;
#3236=ADVANCED_FACE ( 'NONE', ( #4515 ), #1359, .F. ) ;
#3240=CARTESIAN_POINT ( 'NONE',  ( -49.94601516505092320, 87.32303837806215085, -0.6228612347031499130 ) ) ;
#3248=CARTESIAN_POINT ( 'NONE',  ( -49.96742166427387843, 83.19195211451609850, 1.586024383261720239 ) ) ;
#3252=CARTESIAN_POINT ( 'NONE',  ( 41.99613340007108064, 84.41915023570773258, 2.331601159595727779 ) ) ;
#3254=ORIENTED_EDGE ( 'NONE', *, *, #7110, .T. ) ;
#3267=CARTESIAN_POINT ( 'NONE',  ( 41.93355926540186118, 82.63845406065466648, -0.4466446237676945930 ) ) ;
#3288=CARTESIAN_POINT ( 'NONE',  ( -39.83716857408418122, 108.0000000000001990, -4.999999999999976907 ) ) ;
#3300=CARTESIAN_POINT ( 'NONE',  ( -50.00000000000000711, 85.00000000000009948, -2.399999999999999467 ) ) ;
#3301=CARTESIAN_POINT ( 'NONE',  ( 41.97210380486419723, 86.53394040609762783, -1.850206309318216169 ) ) ;
#3302=DIRECTION ( 'NONE',  ( -1.000000000000000000, 0.000000000000000000, 1.412205397084726379E-17 ) ) ;
#3315=DIRECTION ( 'NONE',  ( -1.412205397084881070E-17, 2.775557561562891967E-17, 1.000000000000000000 ) ) ;
#3316=EDGE_CURVE ( 'NONE', #7075, #5556, #1398, .T. ) ;
#3324=CIRCLE ( 'NONE', #4386, 1.250000000000001110 ) ;
#3327=FACE_OUTER_BOUND ( 'NONE', #619, .T. ) ;
#3332=DIRECTION ( 'NONE',  ( -1.000000000000000000, 0.000000000000000000, 0.000000000000000000 ) ) ;
#3339=CARTESIAN_POINT ( 'NONE',  ( 1.270137496355039850E-14, 85.00000000000011369, 5.000000000000046185 ) ) ;
#3344=DIRECTION ( 'NONE',  ( -1.000000000000000000, 0.000000000000000000, 1.112002228190260397E-17 ) ) ;
#3357=ADVANCED_FACE ( 'NONE', ( #3416 ), #6733, .F. ) ;
#3362=CARTESIAN_POINT ( 'NONE',  ( 1.270137496355039850E-14, 85.00000000000011369, 5.000000000000046185 ) ) ;
#3365=CARTESIAN_POINT ( 'NONE',  ( 50.00000000000004974, 85.00000000000039790, -2.399999999999999467 ) ) ;
#3383=CARTESIAN_POINT ( 'NONE',  ( 1.284259550325887758E-14, 85.00000000000005684, -5.000000000000004441 ) ) ;
#3384=FACE_BOUND ( 'NONE', #7180, .T. ) ;
#3392=B_SPLINE_CURVE_WITH_KNOTS ( 'NONE', 3,
 ( #2311, #1103, #4139, #6090, #5392, #3479, #5435, #392, #6003, #2973, #935, #4181, #6754, #2937, #306, #5479, #3518, #2813, #6669, #977, #2348, #4102, #7246, #1016 ),
 .UNSPECIFIED., .F., .F.,
 ( 4, 2, 2, 2, 2, 2, 2, 2, 2, 2, 2, 4 ),
 ( 0.006106748147955515411, 0.006869861680660345471, 0.007632975213365174663, 0.008396088746070003855, 0.009159202278774834782, 0.009540759045127248511, 0.009922315811479663974, 0.01030387257783207944, 0.01068542934418449317, 0.01106698611053690863, 0.01144854287688932409, 0.01221165640959417757 ),
 .UNSPECIFIED. ) ;
#3415=CARTESIAN_POINT ( 'NONE',  ( -41.99800142710427764, 85.46750262719235991, 2.365737336732676610 ) ) ;
#3416=FACE_OUTER_BOUND ( 'NONE', #5623, .T. ) ;
#3421=B_SPLINE_CURVE_WITH_KNOTS ( 'NONE', 3,
 ( #5209, #5243, #1963, #6399, #7099, #7175, #4607, #4030, #703, #3248, #4224, #2149, #979, #6045, #5482, #6756, #308, #2894, #3520, #4721, #2853, #7871, #5394, #2226, #7836, #1065, #3442, #1654, #4141, #7300, #4061, #7957 ),
 .UNSPECIFIED., .F., .F.,
 ( 4, 2, 2, 2, 2, 2, 2, 2, 2, 2, 2, 2, 2, 2, 2, 4 ),
 ( 0.000000000000000000, 0.0004690358444887973298, 0.0009380716889775946596, 0.001407107533466392044, 0.001876143377955189319, 0.002345179222443986595, 0.002814215066932784087, 0.003752286755910362159, 0.004221322600399150977, 0.004690358444887940230, 0.005159394289376728615, 0.005628430133865517868, 0.006097465978354307120, 0.006566501822843097240, 0.007035537667331886492, 0.007504573511820675745 ),
 .UNSPECIFIED. ) ;
#3428=CLOSED_SHELL ( 'NONE', ( #5877, #3236, #6109, #8157, #5270, #1416, #8108, #5444, #3357, #6644, #3515, #5076, #3441, #5200, #1070, #3850, #2457, #7977, #7969, #1270, #2389, #1566, #3812, #7082, #1340, #1553, #1098, #419 ) ) ;
#3429=VECTOR ( 'NONE', #59, 1000.000000000000000 ) ;
#3436=CIRCLE ( 'NONE', #8072, 1.249999999999998002 ) ;
#3441=ADVANCED_FACE ( 'NONE', ( #1764 ), #7890, .T. ) ;
#3442=CARTESIAN_POINT ( 'NONE',  ( -49.98889375043668082, 83.93620601285597616, -2.157108981641785217 ) ) ;
#3444=FACE_OUTER_BOUND ( 'NONE', #4457, .T. ) ;
#3446=CIRCLE ( 'NONE', #1726, 39.00000000000002132 ) ;
#3451=ORIENTED_EDGE ( 'NONE', *, *, #7776, .T. ) ;
#3463=CARTESIAN_POINT ( 'NONE',  ( 1.270137496355039850E-14, 85.00000000000011369, 5.000000000000046185 ) ) ;
#3464=CARTESIAN_POINT ( 'NONE',  ( -41.97904239022133055, 86.32664991614245764, 2.000000000000043521 ) ) ;
#3479=CARTESIAN_POINT ( 'NONE',  ( -41.96864087686231670, 86.63551061574989376, -1.774759388940247984 ) ) ;
#3501=CYLINDRICAL_SURFACE ( 'NONE', #108, 42.00000000000002132 ) ;
#3515=ADVANCED_FACE ( 'NONE', ( #958 ), #3501, .F. ) ;
#3518=CARTESIAN_POINT ( 'NONE',  ( -41.93694813901188212, 87.30092581718484723, 0.6942729367013813491 ) ) ;
#3520=CARTESIAN_POINT ( 'NONE',  ( -49.94812488057640110, 82.72218486298729090, -0.7721950313463720184 ) ) ;
#3535=VECTOR ( 'NONE', #6799, 1000.000000000000000 ) ;
#3540=CARTESIAN_POINT ( 'NONE',  ( 1.270137496355039850E-14, 85.00000000000011369, 5.000000000000046185 ) ) ;
#3544=DIRECTION ( 'NONE',  ( 1.412205397084881070E-17, -2.775557561562891967E-17, -1.000000000000000000 ) ) ;
#3552=EDGE_CURVE ( 'NONE', #493, #1081, #8144, .T. ) ;
#3582=ORIENTED_EDGE ( 'NONE', *, *, #5063, .F. ) ;
#3584=ORIENTED_EDGE ( 'NONE', *, *, #4356, .F. ) ;
#3593=AXIS2_PLACEMENT_3D ( 'NONE', #2753, #6610, #1600 ) ;
#3597=CARTESIAN_POINT ( 'NONE',  ( 42.00000000000003553, 85.23349283444500202, 2.399999999999973266 ) ) ;
#3625=FACE_BOUND ( 'NONE', #6992, .T. ) ;
#3636=CARTESIAN_POINT ( 'NONE',  ( -41.94398068067087593, 82.82972336481591924, 1.056300034359339168 ) ) ;
#3644=DIRECTION ( 'NONE',  ( 1.412205397084881070E-17, -2.775557561562891967E-17, -1.000000000000000000 ) ) ;
#3664=ORIENTED_EDGE ( 'NONE', *, *, #1647, .T. ) ;
#3675=ORIENTED_EDGE ( 'NONE', *, *, #1370, .T. ) ;
#3677=CARTESIAN_POINT ( 'NONE',  ( -41.94165275491890554, 82.78620438794195024, -0.9356232805453277290 ) ) ;
#3683=CARTESIAN_POINT ( 'NONE',  ( 39.83716857408421674, 108.0000000000001421, 4.163336342344337027E-14 ) ) ;
#3690=AXIS2_PLACEMENT_3D ( 'NONE', #3339, #7845, #127 ) ;
#3700=CARTESIAN_POINT ( 'NONE',  ( 49.94236053903781425, 87.40012995604539014, -0.1563225272304197000 ) ) ;
#3714=CIRCLE ( 'NONE', #2002, 39.00000000000002132 ) ;
#3718=CARTESIAN_POINT ( 'NONE',  ( 49.99637462046962355, 84.37866470723844259, -2.323446361670104654 ) ) ;
#3724=ORIENTED_EDGE ( 'NONE', *, *, #5102, .F. ) ;
#3729=CARTESIAN_POINT ( 'NONE',  ( -41.99105870351831982, 84.12501143410540294, -2.238438502733109736 ) ) ;
#3733=DIRECTION ( 'NONE',  ( -1.000000000000000000, 0.000000000000000000, 0.000000000000000000 ) ) ;
#3763=EDGE_CURVE ( 'NONE', #7604, #7241, #5790, .T. ) ;
#3767=CARTESIAN_POINT ( 'NONE',  ( 39.83716857408421674, 108.0000000000001990, -4.999999999999976907 ) ) ;
#3769=ORIENTED_EDGE ( 'NONE', *, *, #4238, .F. ) ;
#3772=CARTESIAN_POINT ( 'NONE',  ( -41.95747712235106519, 83.10910067217422181, -1.483502059617906266 ) ) ;
#3793=CARTESIAN_POINT ( 'NONE',  ( 49.98627395458714062, 86.20659363562862154, 2.098057260256863010 ) ) ;
#3805=CARTESIAN_POINT ( 'NONE',  ( -39.83716857408418122, 108.0000000000001421, 4.163336342344337027E-14 ) ) ;
#3812=ADVANCED_FACE ( 'NONE', ( #7803 ), #1561, .F. ) ;
#3813=CARTESIAN_POINT ( 'NONE',  ( 41.99757081983620566, 85.51235667645809713, -2.358461006662995629 ) ) ;
#3825=CARTESIAN_POINT ( 'NONE',  ( -39.83716857408418122, 108.0000000000001990, -4.999999999999976907 ) ) ;
#3828=ORIENTED_EDGE ( 'NONE', *, *, #6168, .T. ) ;
#3841=ORIENTED_EDGE ( 'NONE', *, *, #7096, .F. ) ;
#3843=DIRECTION ( 'NONE',  ( 0.8571673007021125557, 2.194743421410585277E-16, -0.5150380749100536004 ) ) ;
#3845=DIRECTION ( 'NONE',  ( 1.412205397084881070E-17, -2.775557561562891967E-17, -1.000000000000000000 ) ) ;
#3848=ORIENTED_EDGE ( 'NONE', *, *, #1630, .T. ) ;
#3850=ADVANCED_FACE ( 'NONE', ( #1502 ), #5331, .F. ) ;
#3864=LINE ( 'NONE', #7668, #3429 ) ;
#3869=CARTESIAN_POINT ( 'NONE',  ( -50.00000000000000711, 85.15661249647207853, -2.400000000000023448 ) ) ;
#3872=PRESENTATION_STYLE_ASSIGNMENT (( #6460 ) ) ;
#3886=EDGE_LOOP ( 'NONE', ( #7585, #1911, #5612, #8186 ) ) ;
#3891=B_SPLINE_CURVE_WITH_KNOTS ( 'NONE', 3,
 ( #7729, #6367, #7690, #2552, #3252, #1296, #6942, #1888 ),
 .UNSPECIFIED., .F., .F.,
 ( 4, 2, 2, 4 ),
 ( 0.007505023096728393080, 0.007854877166616045306, 0.008204731236503698399, 0.008904439376279002852 ),
 .UNSPECIFIED. ) ;
#3898=DIRECTION ( 'NONE',  ( 1.000000000000000000, 1.502586498047605218E-16, -1.412205397084881070E-17 ) ) ;
#3901=DIRECTION ( 'NONE',  ( 1.412205397084881070E-17, -2.775557561562891967E-17, -1.000000000000000000 ) ) ;
#3904=CARTESIAN_POINT ( 'NONE',  ( -49.97874610126634565, 86.47445480916303495, -1.919346332466802085 ) ) ;
#3906=LINE ( 'NONE', #696, #5773 ) ;
#3932=CARTESIAN_POINT ( 'NONE',  ( 41.94721337724063659, 82.88985491569346209, -1.171319538143684280 ) ) ;
#3942=CARTESIAN_POINT ( 'NONE',  ( 0.000000000000000000, 0.000000000000000000, 0.000000000000000000 ) ) ;
#3944=CARTESIAN_POINT ( 'NONE',  ( -49.97491191256673915, 86.58758952877983006, 1.806678789609362124 ) ) ;
#3947=CARTESIAN_POINT ( 'NONE',  ( -39.83716857408418122, 108.0000000000001137, 0.7510757737844986348 ) ) ;
#3948=FILL_AREA_STYLE_COLOUR ( '', #4617 ) ;
#3954=VERTEX_POINT ( 'NONE', #2363 ) ;
#3966=CARTESIAN_POINT ( 'NONE',  ( -41.08716857408418122, 108.0000000000001421, 4.161571085597980959E-14 ) ) ;
#3967=CARTESIAN_POINT ( 'NONE',  ( 41.95061225082201162, 87.03752755116852313, -1.274660781186774283 ) ) ;
#3973=EDGE_CURVE ( 'NONE', #7290, #7075, #5025, .T. ) ;
#3978=CONICAL_SURFACE ( 'NONE', #654, 1.250000000000001110, 1.029744258676655200 ) ;
#3979=B_SPLINE_CURVE_WITH_KNOTS ( 'NONE', 3,
 ( #2302, #423, #4837, #6867, #3597, #2964 ),
 .UNSPECIFIED., .F., .F.,
 ( 4, 2, 4 ),
 ( 0.006106730743980896305, 0.006805876920354644692, 0.007505023096728393080 ),
 .UNSPECIFIED. ) ;
#3981=CARTESIAN_POINT ( 'NONE',  ( 42.00000000000003553, 85.00000000000012790, -2.399999999999999023 ) ) ;
#3986=CARTESIAN_POINT ( 'NONE',  ( -49.95669389512426761, 87.08239168930829521, -1.203442334140364389 ) ) ;
#3987=EDGE_LOOP ( 'NONE', ( #5458, #440, #7501, #3584, #1559, #5252 ) ) ;
#3998=CARTESIAN_POINT ( 'NONE',  ( 50.00000000000008527, 84.84140190613213406, -2.399999999999993250 ) ) ;
#4001=ORIENTED_EDGE ( 'NONE', *, *, #4356, .T. ) ;
#4020=CARTESIAN_POINT ( 'NONE',  ( 5.930697612239895941E-15, 38.99999999999999289, -4.999999999999990230 ) ) ;
#4030=CARTESIAN_POINT ( 'NONE',  ( -49.97875682971460520, 83.53682071867368109, 1.908850074583584355 ) ) ;
#4042=EDGE_LOOP ( 'NONE', ( #5816, #1190, #4788 ) ) ;
#4045=CARTESIAN_POINT ( 'NONE',  ( -41.99057649487198063, 85.91769722991278968, 2.230045660306874566 ) ) ;
#4047=DIRECTION ( 'NONE',  ( -1.000000000000000000, 0.000000000000000000, 1.412205397084726379E-17 ) ) ;
#4061=CARTESIAN_POINT ( 'NONE',  ( -50.00000000000000000, 84.84335183244010636, -2.399999999999976374 ) ) ;
#4066=AXIS2_PLACEMENT_3D ( 'NONE', #3805, #7135, #6328 ) ;
#4072=CARTESIAN_POINT ( 'NONE',  ( 50.00000000000003553, 85.00000000000012790, -5.000000000000003553 ) ) ;
#4093=AXIS2_PLACEMENT_3D ( 'NONE', #406, #6638, #2946 ) ;
#4097=VERTEX_POINT ( 'NONE', #155 ) ;
#4098=EDGE_LOOP ( 'NONE', ( #6157, #4911 ) ) ;
#4102=CARTESIAN_POINT ( 'NONE',  ( -41.96465185579608459, 86.73000941357497595, 1.682954651729597018 ) ) ;
#4127=VERTEX_POINT ( 'NONE', #5813 ) ;
#4128=EDGE_CURVE ( 'NONE', #1429, #4916, #3421, .T. ) ;
#4130=CARTESIAN_POINT ( 'NONE',  ( -1.249999999999992673, 38.99999999999999289, -4.999999999999990230 ) ) ;
#4139=CARTESIAN_POINT ( 'NONE',  ( -41.99756812932358940, 85.51244622392444228, -2.358409241415399205 ) ) ;
#4141=CARTESIAN_POINT ( 'NONE',  ( -49.99635120648662934, 84.37668793019695102, -2.322944911472436313 ) ) ;
#4143=CARTESIAN_POINT ( 'NONE',  ( 39.83716857408421674, 108.0000000000001421, 4.163336342344337027E-14 ) ) ;
#4144=ORIENTED_EDGE ( 'NONE', *, *, #7453, .F. ) ;
#4157=SHAPE_DEFINITION_REPRESENTATION ( #6385, #6413 ) ;
#4181=CARTESIAN_POINT ( 'NONE',  ( -41.93162413031724611, 87.39566059415857069, -0.1928755069452474658 ) ) ;
#4193=AXIS2_PLACEMENT_3D ( 'NONE', #872, #1512, #4047 ) ;
#4200=CARTESIAN_POINT ( 'NONE',  ( 1.270137496355039850E-14, 85.00000000000011369, 5.000000000000046185 ) ) ;
#4201=DIRECTION ( 'NONE',  ( 1.412205397084881070E-17, -2.775557561562891967E-17, -1.000000000000000000 ) ) ;
#4202=DIRECTION ( 'NONE',  ( 1.412205397084881070E-17, -2.775557561562891967E-17, -1.000000000000000000 ) ) ;
#4210=CARTESIAN_POINT ( 'NONE',  ( -38.58716857408418122, 108.0000000000001421, 4.165101599090693094E-14 ) ) ;
#4218=VERTEX_POINT ( 'NONE', #1692 ) ;
#4224=CARTESIAN_POINT ( 'NONE',  ( -49.96368263234898421, 83.09261300472543610, 1.465190138156000188 ) ) ;
#4229=CARTESIAN_POINT ( 'NONE',  ( 1.250000000000003997, 38.99999999999999289, -1.765256746356099026E-17 ) ) ;
#4236=CARTESIAN_POINT ( 'NONE',  ( 1.250000000000004663, 38.99999999999999289, -4.999999999999990230 ) ) ;
#4238=EDGE_CURVE ( 'NONE', #5215, #6340, #3050, .T. ) ;
#4244=VECTOR ( 'NONE', #2064, 1000.000000000000000 ) ;
#4262=CARTESIAN_POINT ( 'NONE',  ( -1.249999999999992228, 38.99999999999999289, -1.765256746356098409E-17 ) ) ;
#4277=ORIENTED_EDGE ( 'NONE', *, *, #8164, .T. ) ;
#4289=CARTESIAN_POINT ( 'NONE',  ( 5.860087342385653250E-15, 38.99999999999999289, 0.000000000000000000 ) ) ;
#4308=CARTESIAN_POINT ( 'NONE',  ( -50.00000000000000711, 85.00000000000009948, 5.000000000000047073 ) ) ;
#4309=FACE_OUTER_BOUND ( 'NONE', #6239, .T. ) ;
#4316=DIRECTION ( 'NONE',  ( 1.412205397084881070E-17, -2.775557561562891967E-17, -1.000000000000000000 ) ) ;
#4339=DIRECTION ( 'NONE',  ( -1.000000000000000000, -1.502586498047605218E-16, 1.238733049487200360E-17 ) ) ;
#4344=EDGE_LOOP ( 'NONE', ( #5178, #3196, #3254, #1968 ) ) ;
#4356=EDGE_CURVE ( 'NONE', #1769, #3954, #2975, .T. ) ;
#4363=EDGE_CURVE ( 'NONE', #6955, #910, #1105, .T. ) ;
#4364=CARTESIAN_POINT ( 'NONE',  ( 49.95662654559780691, 87.08399340104908504, -1.200635520122793620 ) ) ;
#4384=ORIENTED_EDGE ( 'NONE', *, *, #3763, .F. ) ;
#4386=AXIS2_PLACEMENT_3D ( 'NONE', #7068, #3086, #6 ) ;
#4426=CARTESIAN_POINT ( 'NONE',  ( 49.95669240716474491, 82.91758674606779778, 1.203334160065640646 ) ) ;
#4430=CARTESIAN_POINT ( 'NONE',  ( 41.93694813901194607, 82.69907418281616174, 0.6942729367014212061 ) ) ;
#4450=DIRECTION ( 'NONE',  ( -1.412205397084881070E-17, 2.775557561562891967E-17, 1.000000000000000000 ) ) ;
#4457=EDGE_LOOP ( 'NONE', ( #3036, #4843, #7731 ) ) ;
#4467=CARTESIAN_POINT ( 'NONE',  ( 41.97907998747123770, 86.32940376908055669, -2.002229301367421055 ) ) ;
#4483=CARTESIAN_POINT ( 'NONE',  ( -49.94237310791755391, 87.39986840612061769, -0.1602877778557319222 ) ) ;
#4514=CARTESIAN_POINT ( 'NONE',  ( 41.93161960896016893, 87.39568130184227357, 0.1926422142524573111 ) ) ;
#4515=FACE_OUTER_BOUND ( 'NONE', #4774, .T. ) ;
#4520=EDGE_CURVE ( 'NONE', #6955, #7075, #1113, .T. ) ;
#4524=DIRECTION ( 'NONE',  ( -1.000000000000000000, 0.000000000000000000, 0.000000000000000000 ) ) ;
#4528=CARTESIAN_POINT ( 'NONE',  ( -49.94311118432959518, 87.38465289139489300, 0.3128412141715384842 ) ) ;
#4531=DIRECTION ( 'NONE',  ( 1.412205397084881070E-17, -2.775557561562891967E-17, -1.000000000000000000 ) ) ;
#4537=ORIENTED_EDGE ( 'NONE', *, *, #4793, .F. ) ;
#4543=CARTESIAN_POINT ( 'NONE',  ( -38.58716857408418122, 108.0000000000001421, 4.161571085597980959E-14 ) ) ;
#4553=CARTESIAN_POINT ( 'NONE',  ( 41.98244464128908504, 86.21953388413311359, -2.071021427375734358 ) ) ;
#4568=DIRECTION ( 'NONE',  ( 1.412205397084881070E-17, -2.775557561562891967E-17, -1.000000000000000000 ) ) ;
#4576=ORIENTED_EDGE ( 'NONE', *, *, #7323, .T. ) ;
#4579=CYLINDRICAL_SURFACE ( 'NONE', #1170, 1.250000000000001110 ) ;
#4584=VERTEX_POINT ( 'NONE', #5343 ) ;
#4597=FACE_BOUND ( 'NONE', #411, .T. ) ;
#4598=CARTESIAN_POINT ( 'NONE',  ( -49.96747517473576750, 86.80656978053563932, -1.587697219280529648 ) ) ;
#4607=CARTESIAN_POINT ( 'NONE',  ( -49.98571321592396544, 83.79770962390497857, 2.083050663831744309 ) ) ;
#4609=CARTESIAN_POINT ( 'NONE',  ( 49.94312129582970528, 82.61555530433814454, 0.3147289805185609635 ) ) ;
#4617=COLOUR_RGB ( '', 0.66274510, 0.83137255, 0.94901961) ;
#4626=VECTOR ( 'NONE', #7183, 1000.000000000000114 ) ;
#4649=AXIS2_PLACEMENT_3D ( 'NONE', #6202, #1056, #3733 ) ;
#4664=ORIENTED_EDGE ( 'NONE', *, *, #3552, .F. ) ;
#4670=CARTESIAN_POINT ( 'NONE',  ( -49.99999999999999289, 85.00000000000005684, 2.400000000000013234 ) ) ;
#4687=DIRECTION ( 'NONE',  ( -1.000000000000000000, 0.000000000000000000, 1.412205397084726379E-17 ) ) ;
#4721=CARTESIAN_POINT ( 'NONE',  ( -49.95346277782373079, 82.84241399044240950, -1.062802698623567466 ) ) ;
#4726=ORIENTED_EDGE ( 'NONE', *, *, #1598, .F. ) ;
#4730=CARTESIAN_POINT ( 'NONE',  ( 1.274374112546295138E-14, 85.00000000000017053, 2.000000000000043521 ) ) ;
#4772=ORIENTED_EDGE ( 'NONE', *, *, #6672, .T. ) ;
#4774=EDGE_LOOP ( 'NONE', ( #6646, #42, #5808, #2001, #57 ) ) ;
#4777=LINE ( 'NONE', #7309, #5425 ) ;
#4788=ORIENTED_EDGE ( 'NONE', *, *, #5024, .F. ) ;
#4793=EDGE_CURVE ( 'NONE', #166, #3060, #3979, .T. ) ;
#4827=ORIENTED_EDGE ( 'NONE', *, *, #667, .F. ) ;
#4837=CARTESIAN_POINT ( 'NONE',  ( 41.99060366484418694, 85.91597045152531109, 2.230540027468066899 ) ) ;
#4843=ORIENTED_EDGE ( 'NONE', *, *, #5499, .T. ) ;
#4865=VECTOR ( 'NONE', #5478, 1000.000000000000114 ) ;
#4911=ORIENTED_EDGE ( 'NONE', *, *, #6302, .T. ) ;
#4912=VECTOR ( 'NONE', #2025, 1000.000000000000000 ) ;
#4916=VERTEX_POINT ( 'NONE', #3300 ) ;
#4928=CIRCLE ( 'NONE', #2396, 50.00000000000002132 ) ;
#4933=CARTESIAN_POINT ( 'NONE',  ( -41.93354940223068894, 82.63827966896762689, -0.4455622145786132249 ) ) ;
#4955=DIRECTION ( 'NONE',  ( 1.000000000000000000, 0.000000000000000000, -2.065146995210483462E-17 ) ) ;
#4959=ORIENTED_EDGE ( 'NONE', *, *, #5063, .T. ) ;
#4960=EDGE_CURVE ( 'NONE', #5220, #6466, #1267, .T. ) ;
#4962=DIRECTION ( 'NONE',  ( 1.412205397084880761E-17, 2.775557561562891967E-17, 1.000000000000000000 ) ) ;
#4963=LINE ( 'NONE', #1672, #2918 ) ;
#4997=VERTEX_POINT ( 'NONE', #1861 ) ;
#5007=CARTESIAN_POINT ( 'NONE',  ( 49.99423685432767428, 84.22705925652886094, 2.277573141052954053 ) ) ;
#5014=( NAMED_UNIT ( * ) SI_UNIT ( $, .STERADIAN. ) SOLID_ANGLE_UNIT ( ) );
#5015=CARTESIAN_POINT ( 'NONE',  ( 60.00000000000004263, 85.00000000000051159, -1.387778780781445676E-14 ) ) ;
#5021=FACE_OUTER_BOUND ( 'NONE', #7865, .T. ) ;
#5024=EDGE_CURVE ( 'NONE', #7730, #4218, #659, .T. ) ;
#5025=B_SPLINE_CURVE_WITH_KNOTS ( 'NONE', 3,
 ( #5576, #428, #6939, #3121, #1834, #3793, #2493, #6275, #1251, #6314, #6848, #5658, #578, #8172, #3164, #3700, #1756, #3213, #5699, #6359, #4364, #6894, #2548, #3079, #666, #6808, #5038, #7566, #1926, #5745 ),
 .UNSPECIFIED., .F., .F.,
 ( 4, 2, 2, 2, 2, 2, 2, 2, 2, 2, 2, 2, 2, 2, 4 ),
 ( 0.007504573511820881310, 0.007973502549960435198, 0.008442431588099987352, 0.009380289664379093395, 0.009849218702518631671, 0.01031814774065816995, 0.01078707677879770822, 0.01125600581693724650, 0.01172493485507678478, 0.01219386389321632305, 0.01266279293135586133, 0.01313172196949539960, 0.01360065100763493788, 0.01406958004577447789, 0.01500743812205355444 ),
 .UNSPECIFIED. ) ;
#5038=CARTESIAN_POINT ( 'NONE',  ( 49.98886144361676287, 86.06516230458066730, -2.156352803700544385 ) ) ;
#5039=ORIENTED_EDGE ( 'NONE', *, *, #5399, .F. ) ;
#5045=AXIS2_PLACEMENT_3D ( 'NONE', #3383, #3315, #7634 ) ;
#5046=CARTESIAN_POINT ( 'NONE',  ( -42.00000000000000711, 85.00000000000011369, 5.000000000000047073 ) ) ;
#5063=EDGE_CURVE ( 'NONE', #6340, #5215, #2386, .T. ) ;
#5076=ADVANCED_FACE ( 'NONE', ( #7854 ), #913, .T. ) ;
#5078=CARTESIAN_POINT ( 'NONE',  ( 1.274374112546295138E-14, 85.00000000000017053, 2.000000000000043521 ) ) ;
#5082=CARTESIAN_POINT ( 'NONE',  ( -49.95352446852410822, 87.15616155047288771, -1.065671633021394449 ) ) ;
#5102=EDGE_CURVE ( 'NONE', #4584, #7616, #3194, .T. ) ;
#5106=VERTEX_POINT ( 'NONE', #956 ) ;
#5108=CARTESIAN_POINT ( 'NONE',  ( 41.93122500247567075, 87.40257814072478482, -0.06338927685536475953 ) ) ;
#5111=DIRECTION ( 'NONE',  ( -1.412205397084881070E-17, 2.775557561562891967E-17, 1.000000000000000000 ) ) ;
#5120=CARTESIAN_POINT ( 'NONE',  ( -49.99637443241779522, 85.62167278847331886, -2.323444847100760491 ) ) ;
#5129=VERTEX_POINT ( 'NONE', #3966 ) ;
#5131=DIRECTION ( 'NONE',  ( 1.412205397084881070E-17, -2.775557561562891967E-17, -1.000000000000000000 ) ) ;
#5145=CARTESIAN_POINT ( 'NONE',  ( 41.93694480353849485, 87.30099207916882165, 0.6941923800780209763 ) ) ;
#5148=DIRECTION ( 'NONE',  ( -1.412205397084881070E-17, 2.775557561562891967E-17, 1.000000000000000000 ) ) ;
#5152=DIRECTION ( 'NONE',  ( 0.000000000000000000, 0.000000000000000000, 1.000000000000000000 ) ) ;
#5160=VECTOR ( 'NONE', #6604, 1000.000000000000000 ) ;
#5174=DIRECTION ( 'NONE',  ( 1.412205397084881070E-17, -2.775557561562891967E-17, -1.000000000000000000 ) ) ;
#5178=ORIENTED_EDGE ( 'NONE', *, *, #150, .F. ) ;
#5182=ADVANCED_BREP_SHAPE_REPRESENTATION ( '', ( #6686, #1587 ), #1249 ) ;
#5186=CARTESIAN_POINT ( 'NONE',  ( 41.94165275491891265, 87.21379561205887399, -0.9356232805456338175 ) ) ;
#5191=AXIS2_PLACEMENT_3D ( 'NONE', #6600, #2795, #3344 ) ;
#5200=ADVANCED_FACE ( 'NONE', ( #5462, #3625 ), #8053, .T. ) ;
#5201=EDGE_CURVE ( 'NONE', #3227, #2013, #3714, .T. ) ;
#5209=CARTESIAN_POINT ( 'NONE',  ( -49.99999999999999289, 85.00000000000005684, 2.400000000000013234 ) ) ;
#5215=VERTEX_POINT ( 'NONE', #6728 ) ;
#5217=CARTESIAN_POINT ( 'NONE',  ( -1.249999999999992228, 38.99999999999999289, 1.765256746356098409E-17 ) ) ;
#5220=VERTEX_POINT ( 'NONE', #1164 ) ;
#5225=CARTESIAN_POINT ( 'NONE',  ( 41.93238906222617146, 82.61770977831005780, 0.3178396967579638077 ) ) ;
#5234=CARTESIAN_POINT ( 'NONE',  ( -49.99926415638493893, 85.31227754079897352, -2.384817760534238218 ) ) ;
#5243=CARTESIAN_POINT ( 'NONE',  ( -50.00000000000000000, 84.84140190613180721, 2.399999999999987921 ) ) ;
#5252=ORIENTED_EDGE ( 'NONE', *, *, #201, .F. ) ;
#5253=UNCERTAINTY_MEASURE_WITH_UNIT (LENGTH_MEASURE( 1.000000000000000082E-05 ), #2108, 'distance_accuracy_value', 'NONE');
#5264=CARTESIAN_POINT ( 'NONE',  ( 1.284259550325887758E-14, 85.00000000000005684, -5.000000000000004441 ) ) ;
#5270=ADVANCED_FACE ( 'NONE', ( #7444 ), #7285, .F. ) ;
#5271=SURFACE_SIDE_STYLE ('',( #5887 ) ) ;
#5278=CARTESIAN_POINT ( 'NONE',  ( 49.99923958211703479, 84.68425784446333182, 2.384302390493924673 ) ) ;
#5286=MECHANICAL_DESIGN_GEOMETRIC_PRESENTATION_REPRESENTATION('',(#213),#94);
#5302=AXIS2_PLACEMENT_3D ( 'NONE', #8083, #6926, #6964 ) ;
#5307=FACE_OUTER_BOUND ( 'NONE', #1447, .T. ) ;
#5319=DIRECTION ( 'NONE',  ( 1.412205397084881070E-17, -2.775557561562891967E-17, -1.000000000000000000 ) ) ;
#5324=EDGE_CURVE ( 'NONE', #1081, #5786, #3324, .T. ) ;
#5331=CYLINDRICAL_SURFACE ( 'NONE', #3690, 42.00000000000002132 ) ;
#5343=CARTESIAN_POINT ( 'NONE',  ( -39.00000000000000711, 85.00000000000017053, 2.000000000000043077 ) ) ;
#5345=DIRECTION ( 'NONE',  ( 0.000000000000000000, 0.000000000000000000, 1.000000000000000000 ) ) ;
#5355=DIRECTION ( 'NONE',  ( 1.412205397084881070E-17, -2.775557561562891967E-17, -1.000000000000000000 ) ) ;
#5357=EDGE_CURVE ( 'NONE', #5862, #4997, #7967, .T. ) ;
#5374=DIRECTION ( 'NONE',  ( -1.000000000000000000, 0.000000000000000000, 0.000000000000000000 ) ) ;
#5382=CARTESIAN_POINT ( 'NONE',  ( -39.83716857408418122, 108.0000000000001421, 4.163336342344337027E-14 ) ) ;
#5392=CARTESIAN_POINT ( 'NONE',  ( -41.98256188053843374, 86.22727746334254562, -2.078089480949581791 ) ) ;
#5394=CARTESIAN_POINT ( 'NONE',  ( -49.96737414687251544, 83.19055800108179710, -1.584620125916080369 ) ) ;
#5399=EDGE_CURVE ( 'NONE', #479, #7219, #7028, .T. ) ;
#5417=ORIENTED_EDGE ( 'NONE', *, *, #5201, .T. ) ;
#5418=FACE_OUTER_BOUND ( 'NONE', #6210, .T. ) ;
#5424=DIRECTION ( 'NONE',  ( 1.412205397084880761E-17, 2.775557561562891967E-17, 1.000000000000000000 ) ) ;
#5425=VECTOR ( 'NONE', #1622, 1000.000000000000000 ) ;
#5430=ORIENTED_EDGE ( 'NONE', *, *, #7037, .T. ) ;
#5435=CARTESIAN_POINT ( 'NONE',  ( -41.96090147793647418, 86.81773748145498359, -1.587618400554034359 ) ) ;
#5442=VECTOR ( 'NONE', #3216, 1000.000000000000000 ) ;
#5444=ADVANCED_FACE ( 'NONE', ( #1892 ), #4579, .F. ) ;
#5458=ORIENTED_EDGE ( 'NONE', *, *, #7301, .F. ) ;
#5462=FACE_OUTER_BOUND ( 'NONE', #4098, .T. ) ;
#5471=DIRECTION ( 'NONE',  ( 1.412205397084881070E-17, -2.775557561562891967E-17, -1.000000000000000000 ) ) ;
#5478=DIRECTION ( 'NONE',  ( 0.8571673007021125557, 2.194743421410585277E-16, -0.5150380749100536004 ) ) ;
#5479=CARTESIAN_POINT ( 'NONE',  ( -41.93504501509995919, 87.33507146524520692, 0.5690079308734952157 ) ) ;
#5482=CARTESIAN_POINT ( 'NONE',  ( -49.94237215279110131, 82.60011171831004617, 0.3139783802610798258 ) ) ;
#5499=EDGE_CURVE ( 'NONE', #4127, #493, #1536, .T. ) ;
#5511=SHAPE_REPRESENTATION_RELATIONSHIP ( 'NONE' , 'NONE' ,  #6413, #5182 ) ;
#5515=ORIENTED_EDGE ( 'NONE', *, *, #7516, .T. ) ;
#5517=FACE_OUTER_BOUND ( 'NONE', #3073, .T. ) ;
#5519=CARTESIAN_POINT ( 'NONE',  ( -42.00000000000000711, 85.00000000000011369, 5.000000000000047073 ) ) ;
#5532=VECTOR ( 'NONE', #7839, 1000.000000000000000 ) ;
#5548=CARTESIAN_POINT ( 'NONE',  ( -41.93162583688302902, 82.60437000624546044, -0.1928873818977043519 ) ) ;
#5554=AXIS2_PLACEMENT_3D ( 'NONE', #7991, #3644, #2851 ) ;
#5556=VERTEX_POINT ( 'NONE', #4072 ) ;
#5576=CARTESIAN_POINT ( 'NONE',  ( 50.00000000000003553, 85.00000000000012790, 2.399999999999971489 ) ) ;
#5579=AXIS2_PLACEMENT_3D ( 'NONE', #6855, #4962, #1671 ) ;
#5594=ORIENTED_EDGE ( 'NONE', *, *, #2930, .T. ) ;
#5604=LINE ( 'NONE', #4308, #7140 ) ;
#5606=DIRECTION ( 'NONE',  ( 1.412205397084881070E-17, -2.775557561562891967E-17, -1.000000000000000000 ) ) ;
#5612=ORIENTED_EDGE ( 'NONE', *, *, #7077, .T. ) ;
#5614=DIRECTION ( 'NONE',  ( 1.000000000000000000, 1.502586498047605218E-16, -1.412205397084881070E-17 ) ) ;
#5623=EDGE_LOOP ( 'NONE', ( #930, #2231, #3664 ) ) ;
#5626=CARTESIAN_POINT ( 'NONE',  ( -42.00000000000000000, 84.76402542465484657, 2.400000000000002576 ) ) ;
#5630=CARTESIAN_POINT ( 'NONE',  ( 50.00000000000003553, 85.00000000000012790, 2.399999999999971489 ) ) ;
#5638=CARTESIAN_POINT ( 'NONE',  ( -41.95061225082201162, 82.96247244883227268, -1.274660781186474745 ) ) ;
#5658=CARTESIAN_POINT ( 'NONE',  ( 49.94817596271298044, 87.27669880683390602, 0.7754554817173049397 ) ) ;
#5662=EDGE_LOOP ( 'NONE', ( #5039, #5594, #1687 ) ) ;
#5671=CARTESIAN_POINT ( 'NONE',  ( 49.96363327394941933, 83.09135878423523991, 1.463402463581969348 ) ) ;
#5676=B_SPLINE_CURVE_WITH_KNOTS ( 'NONE', 3,
 ( #5796, #5723, #2637, #3231, #8190, #5145, #7661, #2059, #4514, #5108, #7041, #6957, #89, #1310, #5186, #7625, #3967, #7705, #2517, #750, #3301, #4467, #4553, #7079, #798, #3813, #5837, #1944 ),
 .UNSPECIFIED., .F., .F.,
 ( 4, 2, 2, 2, 2, 2, 2, 2, 2, 2, 2, 2, 2, 4 ),
 ( 0.000000000000000000, 0.0007633435184945318005, 0.001526687036989063601, 0.001908358796236322291, 0.002290030555483581198, 0.002671702314730840105, 0.003053374073978099446, 0.003435045833225358353, 0.003816717592472616827, 0.004198389351719875734, 0.004580061110967133774, 0.004961732870214391813, 0.005343404629461648986, 0.006106748147956165065 ),
 .UNSPECIFIED. ) ;
#5699=CARTESIAN_POINT ( 'NONE',  ( 49.94811673897446269, 87.27799541866322386, -0.7717081223119550693 ) ) ;
#5703=EDGE_CURVE ( 'NONE', #3085, #5556, #1569, .T. ) ;
#5717=DIRECTION ( 'NONE',  ( 1.412205397084881070E-17, -2.775557561562891967E-17, -1.000000000000000000 ) ) ;
#5723=CARTESIAN_POINT ( 'NONE',  ( 41.97224725382100274, 86.54166769553343386, 1.857373340501009107 ) ) ;
#5741=DIRECTION ( 'NONE',  ( -1.412205397084881070E-17, 2.775557561562891967E-17, 1.000000000000000000 ) ) ;
#5745=CARTESIAN_POINT ( 'NONE',  ( 50.00000000000004974, 85.00000000000039790, -2.399999999999999467 ) ) ;
#5750=ORIENTED_EDGE ( 'NONE', *, *, #1737, .F. ) ;
#5763=CARTESIAN_POINT ( 'NONE',  ( 41.94437084781012715, 82.83815445687697832, 1.050092974071257235 ) ) ;
#5773=VECTOR ( 'NONE', #8167, 1000.000000000000000 ) ;
#5777=FILL_AREA_STYLE ('',( #3948 ) ) ;
#5785=EDGE_CURVE ( 'NONE', #3954, #910, #2104, .T. ) ;
#5786=VERTEX_POINT ( 'NONE', #3162 ) ;
#5789=LINE ( 'NONE', #2017, #2126 ) ;
#5790=LINE ( 'NONE', #5217, #8063 ) ;
#5794=ORIENTED_EDGE ( 'NONE', *, *, #820, .F. ) ;
#5796=CARTESIAN_POINT ( 'NONE',  ( 41.97904239022138029, 86.32664991614251448, 2.000000000000043521 ) ) ;
#5808=ORIENTED_EDGE ( 'NONE', *, *, #4128, .F. ) ;
#5813=CARTESIAN_POINT ( 'NONE',  ( 39.83716857408421674, 108.0000000000001137, 0.7510757737844986348 ) ) ;
#5816=ORIENTED_EDGE ( 'NONE', *, *, #716, .F. ) ;
#5818=CARTESIAN_POINT ( 'NONE',  ( 1.270137496355039850E-14, 85.00000000000011369, 5.000000000000046185 ) ) ;
#5829=AXIS2_PLACEMENT_3D ( 'NONE', #6139, #4316, #6843 ) ;
#5830=ORIENTED_EDGE ( 'NONE', *, *, #5024, .T. ) ;
#5837=CARTESIAN_POINT ( 'NONE',  ( 42.00000000000004263, 85.25453321192475187, -2.400000000000038991 ) ) ;
#5859=CARTESIAN_POINT ( 'NONE',  ( 49.96742166427393528, 83.19195211451632588, -1.586024383261910309 ) ) ;
#5862=VERTEX_POINT ( 'NONE', #6543 ) ;
#5877=ADVANCED_FACE ( 'NONE', ( #2661 ), #2725, .T. ) ;
#5883=COLOUR_RGB ( '', 0.66274510, 0.83137255, 0.94901961) ;
#5887=SURFACE_STYLE_FILL_AREA ( #5777 ) ;
#5894=CARTESIAN_POINT ( 'NONE',  ( 49.98566918070729770, 83.79593159430160654, 2.081985610399850195 ) ) ;
#5970=CARTESIAN_POINT ( 'NONE',  ( -59.99999999999999289, 85.00000000000045475, -2.399999999999999467 ) ) ;
#6003=CARTESIAN_POINT ( 'NONE',  ( -41.94112359463809270, 87.22431328320553234, -0.9366119428082910758 ) ) ;
#6030=EDGE_CURVE ( 'NONE', #1769, #4218, #3392, .T. ) ;
#6032=DIRECTION ( 'NONE',  ( -1.000000000000000000, 0.000000000000000000, 0.000000000000000000 ) ) ;
#6044=FACE_OUTER_BOUND ( 'NONE', #5662, .T. ) ;
#6045=CARTESIAN_POINT ( 'NONE',  ( -49.94550380033327031, 82.66312158132822674, 0.6298752594700357532 ) ) ;
#6051=B_SPLINE_CURVE_WITH_KNOTS ( 'NONE', 3,
 ( #2026, #19, #7115, #6334, #638, #1904, #6382, #3932, #1432, #55, #3267, #1358, #138, #1981, #5225, #2678, #4430, #3189, #5763, #685, #6419, #6449, #1268, #720 ),
 .UNSPECIFIED., .F., .F.,
 ( 4, 2, 2, 2, 2, 2, 2, 2, 2, 2, 2, 4 ),
 ( 0.006106748147956165065, 0.006869861680660866755, 0.007632975213365568445, 0.008396088746070271003, 0.009159202278774973560, 0.009540759045127317900, 0.009922315811479662240, 0.01030387257783200658, 0.01068542934418435265, 0.01106698611053669699, 0.01144854287688904307, 0.01221165640959370746 ),
 .UNSPECIFIED. ) ;
#6057=EDGE_CURVE ( 'NONE', #6897, #6466, #1444, .T. ) ;
#6070=ORIENTED_EDGE ( 'NONE', *, *, #4238, .T. ) ;
#6090=CARTESIAN_POINT ( 'NONE',  ( -41.98889744358045562, 85.99540011155023933, -2.198607263777251575 ) ) ;
#6097=ORIENTED_EDGE ( 'NONE', *, *, #3763, .T. ) ;
#6109=ADVANCED_FACE ( 'NONE', ( #5517 ), #1742, .F. ) ;
#6112=ORIENTED_EDGE ( 'NONE', *, *, #6126, .T. ) ;
#6118=UNCERTAINTY_MEASURE_WITH_UNIT (LENGTH_MEASURE( 1.000000000000000082E-05 ), #1271, 'distance_accuracy_value', 'NONE');
#6121=ORIENTED_EDGE ( 'NONE', *, *, #5102, .T. ) ;
#6126=EDGE_CURVE ( 'NONE', #4097, #1429, #5604, .T. ) ;
#6139=CARTESIAN_POINT ( 'NONE',  ( 1.274374112546295138E-14, 85.00000000000017053, 2.000000000000043521 ) ) ;
#6146=EDGE_LOOP ( 'NONE', ( #6316, #3841, #5515, #4959 ) ) ;
#6156=CARTESIAN_POINT ( 'NONE',  ( 39.83716857408421674, 108.0000000000001990, -4.999999999999976907 ) ) ;
#6157=ORIENTED_EDGE ( 'NONE', *, *, #1350, .T. ) ;
#6161=CARTESIAN_POINT ( 'NONE',  ( -41.93505285506407887, 82.66506966722154459, 0.5694876689910105538 ) ) ;
#6165=ORIENTED_EDGE ( 'NONE', *, *, #4520, .F. ) ;
#6168=EDGE_CURVE ( 'NONE', #4218, #166, #2102, .T. ) ;
#6172=CARTESIAN_POINT ( 'NONE',  ( 42.00000000000003553, 85.00000000000012790, -5.000000000000003553 ) ) ;
#6191=DIRECTION ( 'NONE',  ( -1.000000000000000000, 0.000000000000000000, 2.224004456380520794E-17 ) ) ;
#6197=EDGE_LOOP ( 'NONE', ( #2941, #2746, #2920, #518, #4001, #1048 ) ) ;
#6202=CARTESIAN_POINT ( 'NONE',  ( -39.83716857408418122, 108.0000000000001990, -4.999999999999976907 ) ) ;
#6206=AXIS2_PLACEMENT_3D ( 'NONE', #3362, #4568, #7754 ) ;
#6210=EDGE_LOOP ( 'NONE', ( #3020, #2527, #2670 ) ) ;
#6218=CARTESIAN_POINT ( 'NONE',  ( 41.08716857408421674, 108.0000000000001990, -4.999999999999976907 ) ) ;
#6222=ORIENTED_EDGE ( 'NONE', *, *, #3316, .T. ) ;
#6228=DIRECTION ( 'NONE',  ( -1.412205397084881070E-17, 2.775557561562891967E-17, 1.000000000000000000 ) ) ;
#6229=CARTESIAN_POINT ( 'NONE',  ( 1.284259550325887758E-14, 85.00000000000005684, -5.000000000000004441 ) ) ;
#6239=EDGE_LOOP ( 'NONE', ( #993, #2267, #7267 ) ) ;
#6251=CARTESIAN_POINT ( 'NONE',  ( -42.00000000000000711, 85.00000000000011369, -2.399999999999999911 ) ) ;
#6275=CARTESIAN_POINT ( 'NONE',  ( 49.96747517473578881, 86.80656978053562511, 1.587697219280558958 ) ) ;
#6285=ORIENTED_EDGE ( 'NONE', *, *, #6030, .T. ) ;
#6286=CARTESIAN_POINT ( 'NONE',  ( 49.98887975752123936, 83.93556181870177113, -2.156785159512917716 ) ) ;
#6295=SURFACE_STYLE_USAGE ( .BOTH. , #425 ) ;
#6298=EDGE_CURVE ( 'NONE', #7616, #3227, #3864, .T. ) ;
#6302=EDGE_CURVE ( 'NONE', #5106, #4097, #231, .T. ) ;
#6303=CARTESIAN_POINT ( 'NONE',  ( -1.249999999999992895, 38.99999999999999289, -4.999999999999990230 ) ) ;
#6314=CARTESIAN_POINT ( 'NONE',  ( 49.95669389512431025, 87.08239168930832363, 1.203442334140423231 ) ) ;
#6316=ORIENTED_EDGE ( 'NONE', *, *, #7776, .F. ) ;
#6324=CARTESIAN_POINT ( 'NONE',  ( 38.58716857408421674, 108.0000000000001990, -4.999999999999976907 ) ) ;
#6328=DIRECTION ( 'NONE',  ( -1.000000000000000000, 0.000000000000000000, 1.412205397084726379E-17 ) ) ;
#6334=CARTESIAN_POINT ( 'NONE',  ( 41.98889744358049114, 84.00459988845015857, -2.198607263777018872 ) ) ;
#6340=VERTEX_POINT ( 'NONE', #2242 ) ;
#6349=AXIS2_PLACEMENT_3D ( 'NONE', #6229, #1793, #4955 ) ;
#6350=CARTESIAN_POINT ( 'NONE',  ( -49.96738998307156265, 86.80892218194620114, 1.585032901986263454 ) ) ;
#6359=CARTESIAN_POINT ( 'NONE',  ( 49.95346081399738125, 87.15763333356291298, -1.062739361927934612 ) ) ;
#6367=CARTESIAN_POINT ( 'NONE',  ( 42.00000000000003553, 84.88315974372717676, 2.399999999999971489 ) ) ;
#6382=CARTESIAN_POINT ( 'NONE',  ( 41.96090147793651681, 83.18226251854572695, -1.587618400553736597 ) ) ;
#6385=PRODUCT_DEFINITION_SHAPE ( 'NONE', 'NONE',  #1427 ) ;
#6386=CARTESIAN_POINT ( 'NONE',  ( 1.284259550325887758E-14, 85.00000000000005684, -5.000000000000004441 ) ) ;
#6395=CARTESIAN_POINT ( 'NONE',  ( -49.98627395458710510, 86.20659363562862154, -2.098057260256866119 ) ) ;
#6399=CARTESIAN_POINT ( 'NONE',  ( -49.99637462046958092, 84.37866470723815837, 2.323446361670006954 ) ) ;
#6402=ORIENTED_EDGE ( 'NONE', *, *, #1630, .F. ) ;
#6409=CARTESIAN_POINT ( 'NONE',  ( -41.99055603561590289, 84.08175327132279619, 2.229652810622042125 ) ) ;
#6413=SHAPE_REPRESENTATION ( 'mirror holder', ( #1587 ), #1249 ) ;
#6419=CARTESIAN_POINT ( 'NONE',  ( 41.95400501379508285, 83.03335366937368178, 1.381527937806807271 ) ) ;
#6421=DIRECTION ( 'NONE',  ( 0.000000000000000000, 0.000000000000000000, -1.000000000000000000 ) ) ;
#6424=LINE ( 'NONE', #2610, #4244 ) ;
#6428=CARTESIAN_POINT ( 'NONE',  ( -49.96366046868872246, 86.90794461356699685, -1.464368789226978329 ) ) ;
#6433=DIRECTION ( 'NONE',  ( -0.8571673007021125557, -1.430919794933845163E-16, -0.5150380749100536004 ) ) ;
#6438=DIRECTION ( 'NONE',  ( -1.000000000000000000, 0.000000000000000000, 2.224004456380520794E-17 ) ) ;
#6444=EDGE_CURVE ( 'NONE', #3060, #7290, #4777, .T. ) ;
#6445=ORIENTED_EDGE ( 'NONE', *, *, #6949, .F. ) ;
#6449=CARTESIAN_POINT ( 'NONE',  ( 41.96465185579614143, 83.26999058642596196, 1.682954651729509754 ) ) ;
#6454=DIRECTION ( 'NONE',  ( 1.000000000000000000, 0.000000000000000000, 0.000000000000000000 ) ) ;
#6460=SURFACE_STYLE_USAGE ( .BOTH. , #5271 ) ;
#6466=VERTEX_POINT ( 'NONE', #4236 ) ;
#6467=CARTESIAN_POINT ( 'NONE',  ( 49.94812488057642241, 82.72218486298730511, 0.7721950313462304649 ) ) ;
#6474=CARTESIAN_POINT ( 'NONE',  ( 38.58716857408421674, 108.0000000000001421, 4.165101599090693094E-14 ) ) ;
#6491=AXIS2_PLACEMENT_3D ( 'NONE', #5382, #1481, #2841 ) ;
#6502=DIRECTION ( 'NONE',  ( 1.000000000000000000, 1.502586498047605218E-16, -1.412205397084881070E-17 ) ) ;
#6503=CARTESIAN_POINT ( 'NONE',  ( -49.94597403161980509, 87.32391958025807810, 0.6195456578941136438 ) ) ;
#6505=ORIENTED_EDGE ( 'NONE', *, *, #620, .T. ) ;
#6512=CARTESIAN_POINT ( 'NONE',  ( 49.94550380033331294, 82.66312158132835464, -0.6298752594702436980 ) ) ;
#6514=ORIENTED_EDGE ( 'NONE', *, *, #1598, .T. ) ;
#6525=CARTESIAN_POINT ( 'NONE',  ( -41.99999999999998579, 85.23667541621748001, 2.400000000000024336 ) ) ;
#6532=FACE_OUTER_BOUND ( 'NONE', #4344, .T. ) ;
#6543=CARTESIAN_POINT ( 'NONE',  ( -41.97904239022134476, 83.67335008385822448, 2.000000000000043521 ) ) ;
#6560=DIRECTION ( 'NONE',  ( 1.412205397084881070E-17, -2.775557561562891967E-17, -1.000000000000000000 ) ) ;
#6577=CARTESIAN_POINT ( 'NONE',  ( 42.00000000000003553, 85.00000000000049738, 2.399999999999971934 ) ) ;
#6600=CARTESIAN_POINT ( 'NONE',  ( 1.274374112546295138E-14, 85.00000000000017053, 2.000000000000043521 ) ) ;
#6604=DIRECTION ( 'NONE',  ( 1.412205397084881070E-17, -2.775557561562891967E-17, -1.000000000000000000 ) ) ;
#6610=DIRECTION ( 'NONE',  ( 1.412205397084881070E-17, -2.775557561562891967E-17, -1.000000000000000000 ) ) ;
#6611=CONICAL_SURFACE ( 'NONE', #1178, 1.250000000000001110, 1.029744258676655200 ) ;
#6617=PLANE ( 'NONE',  #7958 ) ;
#6620=EDGE_LOOP ( 'NONE', ( #403, #4726 ) ) ;
#6638=DIRECTION ( 'NONE',  ( -1.412205397084881070E-17, 2.775557561562891967E-17, 1.000000000000000000 ) ) ;
#6643=EDGE_LOOP ( 'NONE', ( #4144, #3724 ) ) ;
#6644=ADVANCED_FACE ( 'NONE', ( #3327 ), #152, .F. ) ;
#6646=ORIENTED_EDGE ( 'NONE', *, *, #7278, .T. ) ;
#6660=DIRECTION ( 'NONE',  ( 1.412205397084881070E-17, -2.775557561562891967E-17, -1.000000000000000000 ) ) ;
#6669=CARTESIAN_POINT ( 'NONE',  ( -41.94437084781007030, 87.16184554312398802, 1.050092974071262786 ) ) ;
#6672=EDGE_CURVE ( 'NONE', #7241, #5220, #3436, .T. ) ;
#6676=ORIENTED_EDGE ( 'NONE', *, *, #5703, .F. ) ;
#6686=MANIFOLD_SOLID_BREP ( 'M4 Clearance Hole2', #3428 ) ;
#6693=DIRECTION ( 'NONE',  ( -1.000000000000000000, 0.000000000000000000, 1.112002228190260397E-17 ) ) ;
#6697=CYLINDRICAL_SURFACE ( 'NONE', #2079, 1.250000000000001110 ) ;
#6711=CARTESIAN_POINT ( 'NONE',  ( -59.99999999999999289, 85.00000000000045475, 2.399999999999971489 ) ) ;
#6718=EDGE_LOOP ( 'NONE', ( #5750, #6285, #7739, #2498, #829 ) ) ;
#6725=ORIENTED_EDGE ( 'NONE', *, *, #6298, .F. ) ;
#6728=CARTESIAN_POINT ( 'NONE',  ( -38.58716857408418122, 108.0000000000001990, -4.999999999999976907 ) ) ;
#6733=CONICAL_SURFACE ( 'NONE', #3167, 1.250000000000001110, 1.029744258676655200 ) ;
#6737=ORIENTED_EDGE ( 'NONE', *, *, #6057, .F. ) ;
#6754=CARTESIAN_POINT ( 'NONE',  ( -41.93122696811912675, 87.40254376044632068, -0.06342023833167842461 ) ) ;
#6756=CARTESIAN_POINT ( 'NONE',  ( -49.94236411077203996, 82.59994436935571116, -0.1557065084607691663 ) ) ;
#6778=DIRECTION ( 'NONE',  ( -1.000000000000000000, -2.775557561562890365E-16, 1.734723475976806478E-17 ) ) ;
#6787=CARTESIAN_POINT ( 'NONE',  ( -41.93694480353852327, 82.69900792083214469, 0.6941923800780730458 ) ) ;
#6790=CIRCLE ( 'NONE', #3233, 42.00000000000002132 ) ;
#6794=CARTESIAN_POINT ( 'NONE',  ( 60.00000000000004263, 85.00000000000051159, -1.387778780781445676E-14 ) ) ;
#6799=DIRECTION ( 'NONE',  ( 0.8571673007021118895, 2.194743421410583551E-16, -0.5150380749100549327 ) ) ;
#6808=CARTESIAN_POINT ( 'NONE',  ( 49.98564705169091837, 86.20508806345003450, -2.081488237565429777 ) ) ;
#6812=ORIENTED_EDGE ( 'NONE', *, *, #2070, .T. ) ;
#6814=DIRECTION ( 'NONE',  ( 1.412205397084881070E-17, -2.775557561562891967E-17, -1.000000000000000000 ) ) ;
#6815=CARTESIAN_POINT ( 'NONE',  ( 4.440873302168275031E-15, 38.99999999999999289, 0.7510757737844847570 ) ) ;
#6821=DIRECTION ( 'NONE',  ( -1.000000000000000000, 0.000000000000000000, 0.000000000000000000 ) ) ;
#6823=AXIS2_PLACEMENT_3D ( 'NONE', #7010, #4531, #1333 ) ;
#6826=CARTESIAN_POINT ( 'NONE',  ( 41.08716857408421674, 108.0000000000001421, 4.165101599090693094E-14 ) ) ;
#6835=DIRECTION ( 'NONE',  ( 1.412205397084881070E-17, -2.775557561562891967E-17, -1.000000000000000000 ) ) ;
#6843=DIRECTION ( 'NONE',  ( -1.000000000000000000, 0.000000000000000000, 1.032573497605241731E-17 ) ) ;
#6847=CARTESIAN_POINT ( 'NONE',  ( 1.284259550325887758E-14, 85.00000000000005684, -5.000000000000004441 ) ) ;
#6848=CARTESIAN_POINT ( 'NONE',  ( 49.95352446852413664, 87.15616155047293034, 1.065671633021458842 ) ) ;
#6855=CARTESIAN_POINT ( 'NONE',  ( 1.270137496355039850E-14, 85.00000000000011369, 5.000000000000046185 ) ) ;
#6867=CARTESIAN_POINT ( 'NONE',  ( 41.99796613401628775, 85.46972184547207974, 2.365094516100901156 ) ) ;
#6868=CARTESIAN_POINT ( 'NONE',  ( -41.93506701445380003, 82.66515142059692778, -0.5699281247693004371 ) ) ;
#6870=( NAMED_UNIT ( * ) PLANE_ANGLE_UNIT ( ) SI_UNIT ( $, .RADIAN. ) );
#6872=VECTOR ( 'NONE', #5606, 1000.000000000000000 ) ;
#6894=CARTESIAN_POINT ( 'NONE',  ( 49.96357426530715884, 86.91018610273397371, -1.461418215542109600 ) ) ;
#6897=VERTEX_POINT ( 'NONE', #6303 ) ;
#6899=CIRCLE ( 'NONE', #6491, 1.250000000000001110 ) ;
#6912=CARTESIAN_POINT ( 'NONE',  ( 49.96368263234901974, 83.09261300472560663, -1.465190138156190924 ) ) ;
#6920=CARTESIAN_POINT ( 'NONE',  ( -41.95042219981622367, 82.95369115198531063, 1.280157006458463531 ) ) ;
#6926=DIRECTION ( 'NONE',  ( -1.412205397084881070E-17, 2.775557561562891967E-17, 1.000000000000000000 ) ) ;
#6938=DIRECTION ( 'NONE',  ( 1.000000000000000000, 2.775557561562890365E-16, -1.734723475976806478E-17 ) ) ;
#6939=CARTESIAN_POINT ( 'NONE',  ( 49.99926415638497446, 85.31227754079901615, 2.384817760534212017 ) ) ;
#6942=CARTESIAN_POINT ( 'NONE',  ( 41.98525237464914284, 83.86985196153031552, 2.130344599767619584 ) ) ;
#6943=VECTOR ( 'NONE', #2349, 1000.000000000000000 ) ;
#6949=EDGE_CURVE ( 'NONE', #493, #7254, #3171, .T. ) ;
#6950=STYLED_ITEM ( 'NONE', ( #2519 ), #5182 ) ;
#6955=VERTEX_POINT ( 'NONE', #3981 ) ;
#6957=CARTESIAN_POINT ( 'NONE',  ( 41.93354940223066762, 87.36172033103325418, -0.4455622145788336597 ) ) ;
#6964=DIRECTION ( 'NONE',  ( 1.000000000000000000, 0.000000000000000000, -1.112002228190260397E-17 ) ) ;
#6968=CARTESIAN_POINT ( 'NONE',  ( -49.98564705169090416, 86.20508806344973607, 2.081488237565525701 ) ) ;
#6980=LINE ( 'NONE', #5046, #5442 ) ;
#6992=EDGE_LOOP ( 'NONE', ( #5417, #6505 ) ) ;
#7003=DIRECTION ( 'NONE',  ( 1.412205397084881070E-17, -2.775557561562891967E-17, -1.000000000000000000 ) ) ;
#7010=CARTESIAN_POINT ( 'NONE',  ( 1.270137496355039850E-14, 85.00000000000011369, 5.000000000000046185 ) ) ;
#7028=LINE ( 'NONE', #4543, #2640 ) ;
#7036=ORIENTED_EDGE ( 'NONE', *, *, #338, .T. ) ;
#7037=EDGE_CURVE ( 'NONE', #5106, #7290, #6424, .T. ) ;
#7041=CARTESIAN_POINT ( 'NONE',  ( 41.93162583688302902, 87.39562999375550589, -0.1928873818979062182 ) ) ;
#7048=CARTESIAN_POINT ( 'NONE',  ( 39.83716857408421674, 108.0000000000001421, 4.163336342344337027E-14 ) ) ;
#7052=CARTESIAN_POINT ( 'NONE',  ( -49.95662654559777849, 87.08399340104890030, 1.200635520122923072 ) ) ;
#7055=DIRECTION ( 'NONE',  ( -1.000000000000000000, 0.000000000000000000, 1.412205397084881070E-17 ) ) ;
#7068=CARTESIAN_POINT ( 'NONE',  ( 39.83716857408421674, 108.0000000000001990, -4.999999999999976907 ) ) ;
#7070=DIRECTION ( 'NONE',  ( -1.000000000000000000, 0.000000000000000000, 1.412205397084881070E-17 ) ) ;
#7075=VERTEX_POINT ( 'NONE', #7165 ) ;
#7077=EDGE_CURVE ( 'NONE', #7241, #6897, #2173, .T. ) ;
#7079=CARTESIAN_POINT ( 'NONE',  ( 41.98843075541680037, 85.99227196424216402, -2.189015531278163174 ) ) ;
#7082=ADVANCED_FACE ( 'NONE', ( #296 ), #2758, .F. ) ;
#7089=CARTESIAN_POINT ( 'NONE',  ( -49.99422766321047362, 85.77334557296515527, -2.277359159638559394 ) ) ;
#7096=EDGE_CURVE ( 'NONE', #5129, #7219, #6899, .T. ) ;
#7099=CARTESIAN_POINT ( 'NONE',  ( -49.99422363137627201, 84.22622254513437667, 2.277283319317688015 ) ) ;
#7102=ORIENTED_EDGE ( 'NONE', *, *, #5201, .F. ) ;
#7106=DIRECTION ( 'NONE',  ( 1.412205397084881070E-17, -2.775557561562891967E-17, -1.000000000000000000 ) ) ;
#7110=EDGE_CURVE ( 'NONE', #6466, #6897, #790, .T. ) ;
#7112=AXIS2_PLACEMENT_3D ( 'NONE', #7450, #2334, #1767 ) ;
#7115=CARTESIAN_POINT ( 'NONE',  ( 41.99756812932361072, 84.48755377607589878, -2.358409241415262425 ) ) ;
#7120=CYLINDRICAL_SURFACE ( 'NONE', #3593, 1.250000000000001110 ) ;
#7127=ORIENTED_EDGE ( 'NONE', *, *, #620, .F. ) ;
#7135=DIRECTION ( 'NONE',  ( 1.412205397084881070E-17, -2.775557561562891967E-17, -1.000000000000000000 ) ) ;
#7140=VECTOR ( 'NONE', #1950, 1000.000000000000000 ) ;
#7153=CARTESIAN_POINT ( 'NONE',  ( 1.274374112546295138E-14, 85.00000000000017053, 2.000000000000043521 ) ) ;
#7165=CARTESIAN_POINT ( 'NONE',  ( 50.00000000000004974, 85.00000000000039790, -2.399999999999999467 ) ) ;
#7167=CYLINDRICAL_SURFACE ( 'NONE', #2925, 2.399999999999985256 ) ;
#7175=CARTESIAN_POINT ( 'NONE',  ( -49.98887975752123225, 83.93556181870150112, 2.156785159512773831 ) ) ;
#7180=EDGE_LOOP ( 'NONE', ( #3582, #3769 ) ) ;
#7183=DIRECTION ( 'NONE',  ( -0.8571673007021125557, -1.430919794933845163E-16, -0.5150380749100536004 ) ) ;
#7184=CARTESIAN_POINT ( 'NONE',  ( 5.860087342385653250E-15, 38.99999999999999289, 0.000000000000000000 ) ) ;
#7199=CARTESIAN_POINT ( 'NONE',  ( 5.930697612239895941E-15, 38.99999999999999289, -4.999999999999990230 ) ) ;
#7205=CARTESIAN_POINT ( 'NONE',  ( 38.58716857408421674, 108.0000000000001421, 4.161571085597980959E-14 ) ) ;
#7219=VERTEX_POINT ( 'NONE', #4210 ) ;
#7230=DIRECTION ( 'NONE',  ( 1.412205397084881070E-17, -2.775557561562891967E-17, -1.000000000000000000 ) ) ;
#7237=CIRCLE ( 'NONE', #2868, 1.250000000000001110 ) ;
#7241=VERTEX_POINT ( 'NONE', #4262 ) ;
#7246=CARTESIAN_POINT ( 'NONE',  ( -41.97224931050724450, 86.54160261602827120, 1.857416509361091039 ) ) ;
#7249=DIRECTION ( 'NONE',  ( -1.412205397084880761E-17, -2.775557561562891967E-17, -1.000000000000000000 ) ) ;
#7254=VERTEX_POINT ( 'NONE', #6826 ) ;
#7267=ORIENTED_EDGE ( 'NONE', *, *, #1466, .T. ) ;
#7270=DIRECTION ( 'NONE',  ( 1.412205397084881070E-17, -2.775557561562891967E-17, -1.000000000000000000 ) ) ;
#7278=EDGE_CURVE ( 'NONE', #5862, #1769, #1002, .T. ) ;
#7285=CONICAL_SURFACE ( 'NONE', #128, 1.249999999999998002, 1.029744258676653645 ) ;
#7286=CARTESIAN_POINT ( 'NONE',  ( 38.58716857408421674, 108.0000000000001990, -4.999999999999976907 ) ) ;
#7287=VECTOR ( 'NONE', #6660, 1000.000000000000000 ) ;
#7290=VERTEX_POINT ( 'NONE', #3096 ) ;
#7300=CARTESIAN_POINT ( 'NONE',  ( -49.99923958211701347, 84.68425784446330340, -2.384302390493951762 ) ) ;
#7301=EDGE_CURVE ( 'NONE', #6955, #2355, #6051, .T. ) ;
#7309=CARTESIAN_POINT ( 'NONE',  ( 60.00000000000004263, 85.00000000000051159, 2.399999999999971489 ) ) ;
#7319=DIRECTION ( 'NONE',  ( 1.412205397084881070E-17, -2.775557561562891967E-17, -1.000000000000000000 ) ) ;
#7320=CONICAL_SURFACE ( 'NONE', #2567, 1.250000000000001110, 1.029744258676655200 ) ;
#7323=EDGE_CURVE ( 'NONE', #166, #6955, #5676, .T. ) ;
#7346=EDGE_CURVE ( 'NONE', #4997, #4218, #611, .T. ) ;
#7357=CARTESIAN_POINT ( 'NONE',  ( 1.270137496355039850E-14, 85.00000000000011369, 5.000000000000046185 ) ) ;
#7414=VECTOR ( 'NONE', #5614, 1000.000000000000000 ) ;
#7419=AXIS2_PLACEMENT_3D ( 'NONE', #7153, #285, #202 ) ;
#7421=DIRECTION ( 'NONE',  ( 1.412205397084881070E-17, -2.775557561562891967E-17, -1.000000000000000000 ) ) ;
#7444=FACE_OUTER_BOUND ( 'NONE', #1711, .T. ) ;
#7450=CARTESIAN_POINT ( 'NONE',  ( 1.270137496355039850E-14, 85.00000000000011369, 5.000000000000046185 ) ) ;
#7453=EDGE_CURVE ( 'NONE', #7616, #4584, #1601, .T. ) ;
#7469=LINE ( 'NONE', #4229, #3535 ) ;
#7498=SURFACE_STYLE_FILL_AREA ( #8193 ) ;
#7501=ORIENTED_EDGE ( 'NONE', *, *, #5785, .F. ) ;
#7509=ORIENTED_EDGE ( 'NONE', *, *, #1647, .F. ) ;
#7516=EDGE_CURVE ( 'NONE', #5129, #6340, #4963, .T. ) ;
#7525=CARTESIAN_POINT ( 'NONE',  ( -41.97904239022134476, 83.67335008385822448, 2.000000000000043521 ) ) ;
#7539=FACE_OUTER_BOUND ( 'NONE', #544, .T. ) ;
#7560=AXIS2_PLACEMENT_3D ( 'NONE', #7199, #5471, #1515 ) ;
#7561=CARTESIAN_POINT ( 'NONE',  ( 60.00000000000004263, 85.00000000000051159, -2.399999999999999467 ) ) ;
#7566=CARTESIAN_POINT ( 'NONE',  ( 49.99683717277851258, 85.63216245974612661, -2.336254100262029176 ) ) ;
#7569=AXIS2_PLACEMENT_3D ( 'NONE', #3825, #2350, #8162 ) ;
#7576=AXIS2_PLACEMENT_3D ( 'NONE', #5015, #3898, #6421 ) ;
#7585=ORIENTED_EDGE ( 'NONE', *, *, #4960, .F. ) ;
#7602=CARTESIAN_POINT ( 'NONE',  ( -49.94811673897444848, 87.27799541866311017, 0.7717081223120660916 ) ) ;
#7604=VERTEX_POINT ( 'NONE', #6815 ) ;
#7616=VERTEX_POINT ( 'NONE', #126 ) ;
#7624=CARTESIAN_POINT ( 'NONE',  ( 1.250000000000004441, 38.99999999999999289, -4.999999999999990230 ) ) ;
#7625=CARTESIAN_POINT ( 'NONE',  ( 41.94739886896327619, 87.10210726516650936, -1.165086683815467206 ) ) ;
#7634=DIRECTION ( 'NONE',  ( 1.000000000000000000, 0.000000000000000000, -2.065146995210483462E-17 ) ) ;
#7642=CARTESIAN_POINT ( 'NONE',  ( -41.08716857408418122, 108.0000000000001421, 4.165101599090693094E-14 ) ) ;
#7651=ORIENTED_EDGE ( 'NONE', *, *, #5703, .T. ) ;
#7661=CARTESIAN_POINT ( 'NONE',  ( 41.93505285506405045, 87.33493033277945017, 0.5694876689909349476 ) ) ;
#7664=AXIS2_PLACEMENT_3D ( 'NONE', #721, #4339, #90 ) ;
#7668=CARTESIAN_POINT ( 'NONE',  ( 39.00000000000003553, 85.00000000000017053, 2.000000000000043077 ) ) ;
#7677=CARTESIAN_POINT ( 'NONE',  ( 5.860087342385653250E-15, 38.99999999999999289, 0.000000000000000000 ) ) ;
#7690=CARTESIAN_POINT ( 'NONE',  ( 41.99951245237345177, 84.76684522874218430, 2.391513083590206534 ) ) ;
#7698=AXIS2_PLACEMENT_3D ( 'NONE', #3463, #7270, #7741 ) ;
#7705=CARTESIAN_POINT ( 'NONE',  ( 41.95747712235107940, 86.89089932782653136, -1.483502059618200253 ) ) ;
#7723=AXIS2_PLACEMENT_3D ( 'NONE', #2188, #7249, #2854 ) ;
#7729=CARTESIAN_POINT ( 'NONE',  ( 42.00000000000003553, 85.00000000000049738, 2.399999999999971934 ) ) ;
#7730=VERTEX_POINT ( 'NONE', #744 ) ;
#7731=ORIENTED_EDGE ( 'NONE', *, *, #6949, .T. ) ;
#7736=APPLICATION_CONTEXT ( 'automotive_design' ) ;
#7739=ORIENTED_EDGE ( 'NONE', *, *, #7346, .F. ) ;
#7740=ORIENTED_EDGE ( 'NONE', *, *, #2683, .T. ) ;
#7741=DIRECTION ( 'NONE',  ( -1.000000000000000000, -2.775557561562890365E-16, 1.734723475976806478E-17 ) ) ;
#7743=CARTESIAN_POINT ( 'NONE',  ( 50.00000000000003553, 85.00000000000012790, 5.000000000000045297 ) ) ;
#7754=DIRECTION ( 'NONE',  ( -1.000000000000000000, 0.000000000000000000, 2.065146995210483462E-17 ) ) ;
#7756=ORIENTED_EDGE ( 'NONE', *, *, #7037, .F. ) ;
#7768=EDGE_LOOP ( 'NONE', ( #1265, #6097, #4772 ) ) ;
#7769=CIRCLE ( 'NONE', #4193, 1.250000000000001110 ) ;
#7772=CARTESIAN_POINT ( 'NONE',  ( -42.00000000000000711, 85.00000000000046896, 2.399999999999971045 ) ) ;
#7776=EDGE_CURVE ( 'NONE', #7219, #5215, #5789, .T. ) ;
#7803=FACE_OUTER_BOUND ( 'NONE', #7768, .T. ) ;
#7818=FACE_OUTER_BOUND ( 'NONE', #1800, .T. ) ;
#7821=EDGE_CURVE ( 'NONE', #4997, #1429, #2273, .T. ) ;
#7827=FACE_BOUND ( 'NONE', #6620, .T. ) ;
#7836=CARTESIAN_POINT ( 'NONE',  ( -49.97873132679185915, 83.53599209938492720, -1.908173386893793566 ) ) ;
#7837=PLANE ( 'NONE',  #7723 ) ;
#7839=DIRECTION ( 'NONE',  ( -1.000000000000000000, -1.502586498047605218E-16, 1.238733049487200360E-17 ) ) ;
#7845=DIRECTION ( 'NONE',  ( 1.412205397084881070E-17, -2.775557561562891967E-17, -1.000000000000000000 ) ) ;
#7854=FACE_OUTER_BOUND ( 'NONE', #2308, .T. ) ;
#7855=CARTESIAN_POINT ( 'NONE',  ( 1.274374112546295138E-14, 85.00000000000017053, 2.000000000000043521 ) ) ;
#7865=EDGE_LOOP ( 'NONE', ( #7878, #6121, #1080, #7127 ) ) ;
#7867=CARTESIAN_POINT ( 'NONE',  ( -50.00000000000000711, 85.00000000000009948, -5.000000000000005329 ) ) ;
#7871=CARTESIAN_POINT ( 'NONE',  ( -49.96363327394940512, 83.09135878423528254, -1.463402463582062829 ) ) ;
#7872=FACE_OUTER_BOUND ( 'NONE', #376, .T. ) ;
#7878=ORIENTED_EDGE ( 'NONE', *, *, #2648, .F. ) ;
#7886=ORIENTED_EDGE ( 'NONE', *, *, #6126, .F. ) ;
#7890=CYLINDRICAL_SURFACE ( 'NONE', #2236, 50.00000000000002132 ) ;
#7933=CIRCLE ( 'NONE', #116, 1.249999999999998002 ) ;
#7935=CYLINDRICAL_SURFACE ( 'NONE', #7112, 42.00000000000002132 ) ;
#7957=CARTESIAN_POINT ( 'NONE',  ( -50.00000000000000711, 85.00000000000009948, -2.399999999999999467 ) ) ;
#7958=AXIS2_PLACEMENT_3D ( 'NONE', #5264, #5424, #6502 ) ;
#7967=B_SPLINE_CURVE_WITH_KNOTS ( 'NONE', 3,
 ( #7525, #626, #6409, #1259, #5626, #44 ),
 .UNSPECIFIED., .F., .F.,
 ( 4, 2, 4 ),
 ( 0.01361260127035726804, 0.01431046602193920651, 0.01500833077352114499 ),
 .UNSPECIFIED. ) ;
#7969=ADVANCED_FACE ( 'NONE', ( #6044 ), #3978, .F. ) ;
#7977=ADVANCED_FACE ( 'NONE', ( #5021 ), #1870, .F. ) ;
#7991=CARTESIAN_POINT ( 'NONE',  ( 5.930697612239895941E-15, 38.99999999999999289, -4.999999999999990230 ) ) ;
#8010=ORIENTED_EDGE ( 'NONE', *, *, #7516, .F. ) ;
#8018=UNCERTAINTY_MEASURE_WITH_UNIT (LENGTH_MEASURE( 1.000000000000000082E-05 ), #468, 'distance_accuracy_value', 'NONE');
#8019=ORIENTED_EDGE ( 'NONE', *, *, #1350, .F. ) ;
#8039=ORIENTED_EDGE ( 'NONE', *, *, #3973, .F. ) ;
#8053=PLANE ( 'NONE',  #5579 ) ;
#8063=VECTOR ( 'NONE', #1464, 1000.000000000000000 ) ;
#8072=AXIS2_PLACEMENT_3D ( 'NONE', #7677, #2039, #7055 ) ;
#8083=CARTESIAN_POINT ( 'NONE',  ( 1.274374112546295138E-14, 85.00000000000017053, 2.000000000000043521 ) ) ;
#8108=ADVANCED_FACE ( 'NONE', ( #4309 ), #6611, .F. ) ;
#8114=CARTESIAN_POINT ( 'NONE',  ( -41.98843075541677194, 84.00772803575827652, -2.189015531277937132 ) ) ;
#8144=LINE ( 'NONE', #6324, #766 ) ;
#8152=CARTESIAN_POINT ( 'NONE',  ( -41.97904239022134476, 83.67335008385822448, 2.000000000000043521 ) ) ;
#8157=ADVANCED_FACE ( 'NONE', ( #6532 ), #842, .F. ) ;
#8158=EDGE_LOOP ( 'NONE', ( #2791, #72, #2874 ) ) ;
#8162=DIRECTION ( 'NONE',  ( -1.000000000000000000, 0.000000000000000000, 0.000000000000000000 ) ) ;
#8164=EDGE_CURVE ( 'NONE', #910, #3954, #2905, .T. ) ;
#8167=DIRECTION ( 'NONE',  ( 1.412205397084881070E-17, -2.775557561562891967E-17, -1.000000000000000000 ) ) ;
#8172=CARTESIAN_POINT ( 'NONE',  ( 49.94313152867115235, 87.38422970439145843, 0.3160888171753749032 ) ) ;
#8185=CARTESIAN_POINT ( 'NONE',  ( 49.97498335796547053, 83.41456698278581428, 1.808729786019549923 ) ) ;
#8186=ORIENTED_EDGE ( 'NONE', *, *, #6057, .T. ) ;
#8190=CARTESIAN_POINT ( 'NONE',  ( 41.94398068067085461, 87.17027663518501868, 1.056300034359340723 ) ) ;
#8193=FILL_AREA_STYLE ('',( #3098 ) ) ;
#8202=DIRECTION ( 'NONE',  ( 0.000000000000000000, 0.000000000000000000, -1.000000000000000000 ) ) ;
ENDSEC;
END-ISO-10303-21;
